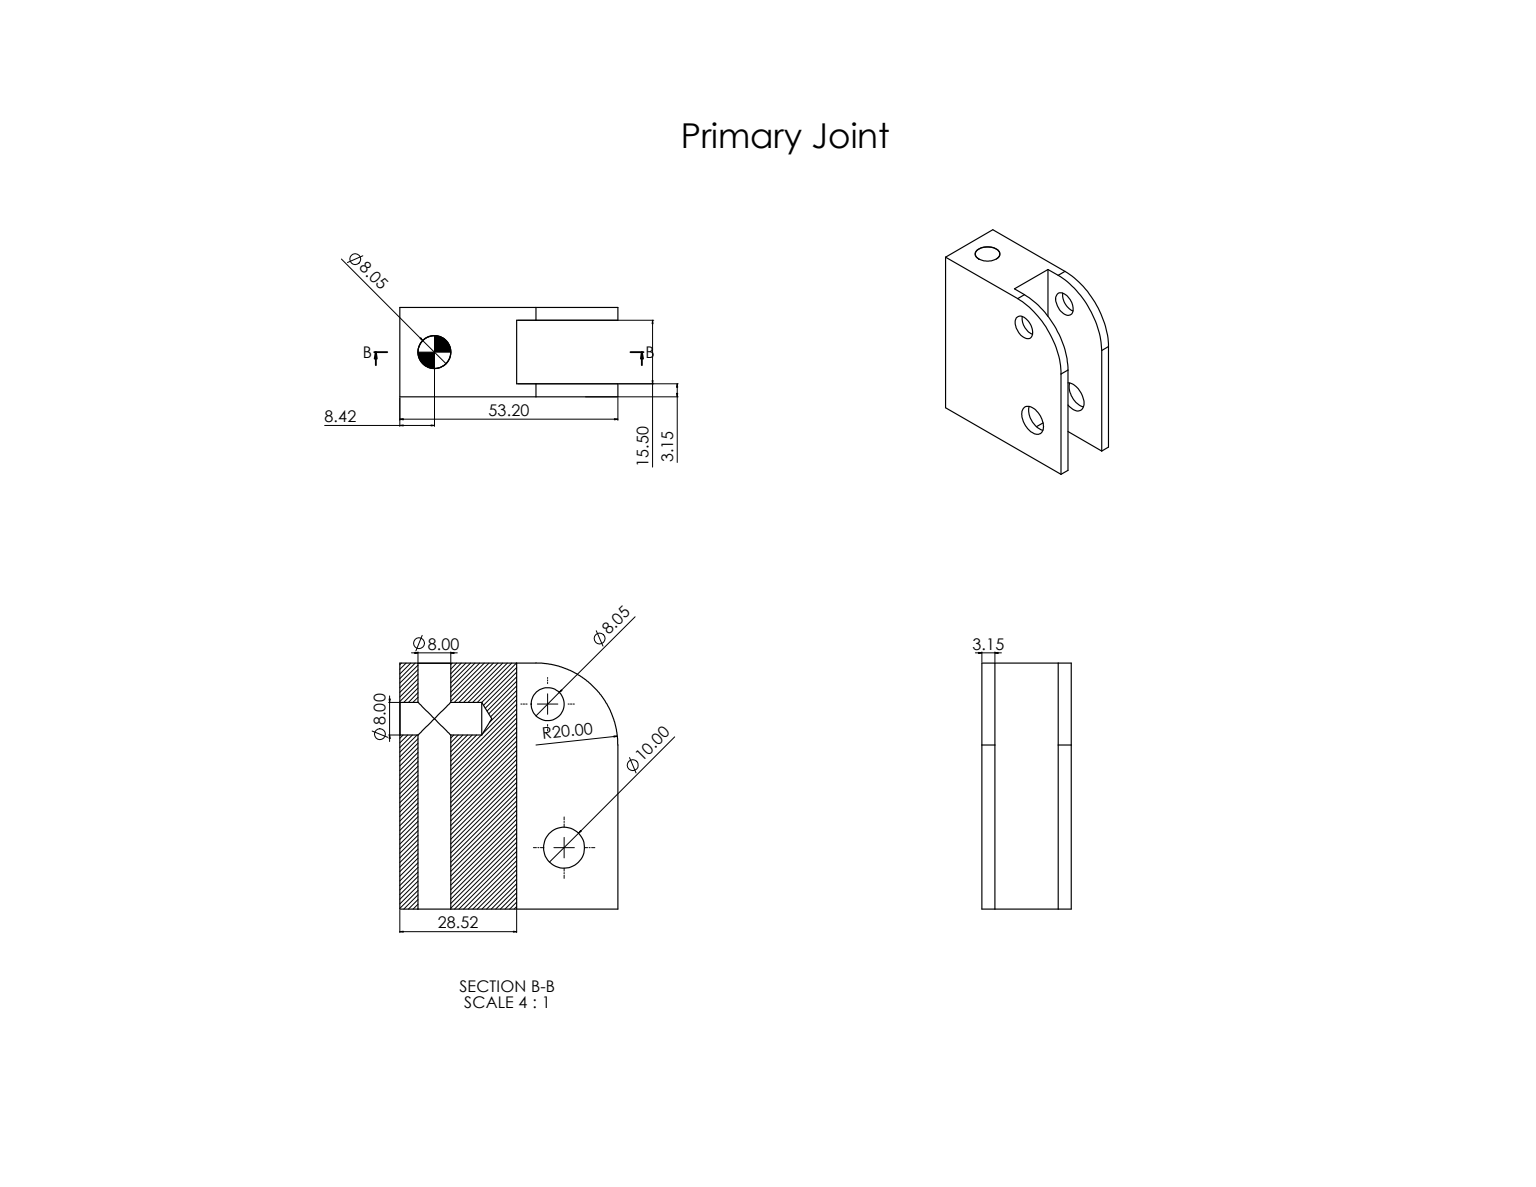
ISO-10303-21;
HEADER;
FILE_DESCRIPTION (('STEP AP214'),
    '1' );
FILE_NAME ('Primary Joint.step',
    '2026-10-20T14:49:59',
    ( '' ),
    ( '' ),
    'SwSTEP 2.0',
    'SolidWorks 2025',
    '' );
FILE_SCHEMA (( 'AUTOMOTIVE_DESIGN' ));
ENDSEC;

DATA;
#6=ORIENTED_EDGE ( 'NONE', *, *, #7618, .F. ) ;
#9=ORIENTED_EDGE ( 'NONE', *, *, #9037, .T. ) ;
#11=CARTESIAN_POINT ( 'NONE',  ( -47.94539818030330025, 137.0132282531173473, 3.999999999999991562 ) ) ;
#12=DIRECTION ( 'NONE',  ( 0.000000000000000000, 0.000000000000000000, 1.000000000000000000 ) ) ;
#20=ORIENTED_EDGE ( 'NONE', *, *, #4444, .T. ) ;
#26=AXIS2_PLACEMENT_3D ( 'NONE', #141, #5845, #6542 ) ;
#28=VECTOR ( 'NONE', #9785, 1000.000000000000000 ) ;
#38=AXIS2_PLACEMENT_3D ( 'NONE', #7742, #2701, #6091 ) ;
#50=DIRECTION ( 'NONE',  ( 1.000000000000000000, 0.000000000000000000, -1.734723475976805615E-16 ) ) ;
#62=ORIENTED_EDGE ( 'NONE', *, *, #3204, .F. ) ;
#63=CARTESIAN_POINT ( 'NONE',  ( -47.94539818030330025, 150.5696653505793563, 3.999999999999993339 ) ) ;
#68=CIRCLE ( 'NONE', #1421, 4.025000000000000355 ) ;
#84=VERTEX_POINT ( 'NONE', #3844 ) ;
#85=DIRECTION ( 'NONE',  ( 0.000000000000000000, 0.000000000000000000, -1.000000000000000000 ) ) ;
#96=DIRECTION ( 'NONE',  ( 0.000000000000000000, 0.000000000000000000, 1.000000000000000000 ) ) ;
#122=ORIENTED_EDGE ( 'NONE', *, *, #3348, .T. ) ;
#134=CIRCLE ( 'NONE', #4024, 3.999999999999993339 ) ;
#140=ORIENTED_EDGE ( 'NONE', *, *, #5070, .F. ) ;
#141=CARTESIAN_POINT ( 'NONE',  ( -23.17384457509314899, 130.5696653505793847, 10.90000000000000036 ) ) ;
#148=FACE_OUTER_BOUND ( 'NONE', #7245, .T. ) ;
#154=AXIS2_PLACEMENT_3D ( 'NONE', #9604, #3022, #736 ) ;
#166=CONICAL_SURFACE ( 'NONE', #1514, 4.025000000000000355, 0.7853981633977258348 ) ;
#168=ADVANCED_FACE ( 'NONE', ( #10363, #4632, #9677 ), #1511, .F. ) ;
#217=ORIENTED_EDGE ( 'NONE', *, *, #8260, .F. ) ;
#231=ORIENTED_EDGE ( 'NONE', *, *, #934, .T. ) ;
#236=DIRECTION ( 'NONE',  ( -1.000000000000000000, 0.000000000000000000, 9.101836848464096770E-17 ) ) ;
#240=EDGE_CURVE ( 'NONE', #10167, #8252, #4254, .T. ) ;
#245=CIRCLE ( 'NONE', #4296, 4.024999999999997691 ) ;
#250=AXIS2_PLACEMENT_3D ( 'NONE', #3199, #920, #4939 ) ;
#254=CARTESIAN_POINT ( 'NONE',  ( -56.36957570605427748, 150.5696653505793563, 10.90000000000000036 ) ) ;
#276=CARTESIAN_POINT ( 'NONE',  ( -21.29350689640810046, 105.5289575273812233, -25.04213562373096380 ) ) ;
#277=AXIS2_PLACEMENT_3D ( 'NONE', #10005, #5118, #7559 ) ;
#281=CARTESIAN_POINT ( 'NONE',  ( -27.85255513972543895, 150.5696653505793563, -7.749999999999996447 ) ) ;
#286=SHAPE_REPRESENTATION ( 'Primary Joint', ( #4601 ), #409 ) ;
#325=AXIS2_PLACEMENT_3D ( 'NONE', #7109, #9549, #7950 ) ;
#331=LINE ( 'NONE', #7790, #7501 ) ;
#343=DIRECTION ( 'NONE',  ( 1.000000000000000000, 0.000000000000000000, -9.101836848464095537E-17 ) ) ;
#350=CARTESIAN_POINT ( 'NONE',  ( -3.173844575093148990, 90.52895752738122326, -7.750000000000000000 ) ) ;
#360=DIRECTION ( 'NONE',  ( -0.000000000000000000, 1.000000000000000000, -0.000000000000000000 ) ) ;
#361=EDGE_LOOP ( 'NONE', ( #8543, #5301 ) ) ;
#374=VECTOR ( 'NONE', #4417, 1000.000000000000000 ) ;
#380=DIRECTION ( 'NONE',  ( -9.101836848464095537E-17, -0.000000000000000000, -1.000000000000000000 ) ) ;
#382=VERTEX_POINT ( 'NONE', #6794 ) ;
#386=AXIS2_PLACEMENT_3D ( 'NONE', #4274, #4902, #96 ) ;
#397=ORIENTED_EDGE ( 'NONE', *, *, #981, .F. ) ;
#404=LINE ( 'NONE', #3533, #7016 ) ;
#407=ORIENTED_EDGE ( 'NONE', *, *, #2639, .F. ) ;
#409=( GEOMETRIC_REPRESENTATION_CONTEXT ( 3 ) GLOBAL_UNCERTAINTY_ASSIGNED_CONTEXT ( ( #7381 ) ) GLOBAL_UNIT_ASSIGNED_CONTEXT ( ( #5955, #7452, #1930 ) ) REPRESENTATION_CONTEXT ( 'NONE', 'WORKASPACE' ) );
#435=CARTESIAN_POINT ( 'NONE',  ( -20.29350689640809691, 140.5696653505793563, -7.749999999999996447 ) ) ;
#445=FACE_OUTER_BOUND ( 'NONE', #4657, .T. ) ;
#459=VECTOR ( 'NONE', #2787, 1000.000000000000000 ) ;
#474=FACE_OUTER_BOUND ( 'NONE', #5248, .T. ) ;
#502=AXIS2_PLACEMENT_3D ( 'NONE', #2591, #6613, #4182 ) ;
#518=DIRECTION ( 'NONE',  ( -0.000000000000000000, 0.000000000000000000, -1.000000000000000000 ) ) ;
#526=PLANE ( 'NONE',  #8406 ) ;
#537=ORIENTED_EDGE ( 'NONE', *, *, #5206, .F. ) ;
#571=ORIENTED_EDGE ( 'NONE', *, *, #1163, .T. ) ;
#593=ORIENTED_EDGE ( 'NONE', *, *, #10466, .T. ) ;
#605=ADVANCED_FACE ( 'NONE', ( #5619 ), #1444, .F. ) ;
#610=DIRECTION ( 'NONE',  ( 0.000000000000000000, 1.000000000000000000, 0.000000000000000000 ) ) ;
#613=ORIENTED_EDGE ( 'NONE', *, *, #690, .T. ) ;
#614=CARTESIAN_POINT ( 'NONE',  ( -47.94539818030330025, 150.5696653505793563, 4.025000000000000355 ) ) ;
#615=EDGE_CURVE ( 'NONE', #2082, #4136, #3892, .T. ) ;
#623=VERTEX_POINT ( 'NONE', #3349 ) ;
#646=APPLICATION_CONTEXT ( 'automotive_design' ) ;
#661=ORIENTED_EDGE ( 'NONE', *, *, #1974, .F. ) ;
#665=LINE ( 'NONE', #3847, #1646 ) ;
#677=EDGE_CURVE ( 'NONE', #4096, #6235, #1697, .T. ) ;
#684=EDGE_LOOP ( 'NONE', ( #10046, #2690, #7813, #7655 ) ) ;
#690=EDGE_CURVE ( 'NONE', #1644, #4219, #1648, .T. ) ;
#691=EDGE_CURVE ( 'NONE', #1746, #382, #7319, .T. ) ;
#692=FACE_OUTER_BOUND ( 'NONE', #7714, .T. ) ;
#697=EDGE_LOOP ( 'NONE', ( #5887, #6931, #9069, #397 ) ) ;
#699=CARTESIAN_POINT ( 'NONE',  ( -36.36957570605426326, 137.0132282531173473, 4.000000000000003553 ) ) ;
#703=DIRECTION ( 'NONE',  ( 1.000000000000000000, 0.000000000000000000, 0.000000000000000000 ) ) ;
#725=LINE ( 'NONE', #4650, #5911 ) ;
#729=CARTESIAN_POINT ( 'NONE',  ( -20.29350689640809691, 140.5696653505793563, 10.90000000000000036 ) ) ;
#736=DIRECTION ( 'NONE',  ( 1.000000000000000000, 0.000000000000000000, 0.000000000000000000 ) ) ;
#744=EDGE_CURVE ( 'NONE', #623, #6132, #1660, .T. ) ;
#769=AXIS2_PLACEMENT_3D ( 'NONE', #8126, #4104, #6540 ) ;
#785=CARTESIAN_POINT ( 'NONE',  ( -3.173844575093148990, 90.52895752738122326, -10.90000000000000036 ) ) ;
#805=EDGE_CURVE ( 'NONE', #4824, #2551, #1327, .T. ) ;
#807=ORIENTED_EDGE ( 'NONE', *, *, #5966, .T. ) ;
#808=DIRECTION ( 'NONE',  ( -1.000000000000000000, 0.000000000000000000, 8.673617379884035472E-17 ) ) ;
#821=LINE ( 'NONE', #4057, #7300 ) ;
#840=CARTESIAN_POINT ( 'NONE',  ( -56.36957570605426326, 90.52895752738122326, -10.90000000000000036 ) ) ;
#841=DIRECTION ( 'NONE',  ( -9.101836848464095537E-17, -0.000000000000000000, -1.000000000000000000 ) ) ;
#854=EDGE_LOOP ( 'NONE', ( #9526, #8200, #20, #9001 ) ) ;
#866=STYLED_ITEM('',(#10532),#9943);
#868=EDGE_CURVE ( 'NONE', #10419, #3877, #1219, .T. ) ;
#877=CARTESIAN_POINT ( 'NONE',  ( -20.29350689640809691, 140.5696653505793563, 10.90000000000000036 ) ) ;
#879=CARTESIAN_POINT ( 'NONE',  ( -11.29350689640809158, 105.5289575273812233, -10.90000000000000036 ) ) ;
#887=LINE ( 'NONE', #2642, #9640 ) ;
#894=EDGE_CURVE ( 'NONE', #8252, #3355, #2912, .T. ) ;
#897=ORIENTED_EDGE ( 'NONE', *, *, #8642, .F. ) ;
#907=VECTOR ( 'NONE', #3811, 1000.000000000000000 ) ;
#920=DIRECTION ( 'NONE',  ( 1.137729606058012035E-16, 0.000000000000000000, 1.000000000000000000 ) ) ;
#923=ORIENTED_EDGE ( 'NONE', *, *, #5411, .F. ) ;
#934=EDGE_CURVE ( 'NONE', #8880, #7785, #4717, .T. ) ;
#950=CARTESIAN_POINT ( 'NONE',  ( -56.36957570605427748, 150.5696653505793563, -10.90000000000000036 ) ) ;
#960=CARTESIAN_POINT ( 'NONE',  ( -47.94539818030330025, 150.5446653505793790, -3.999999999999989786 ) ) ;
#981=EDGE_CURVE ( 'NONE', #2288, #3945, #9975, .T. ) ;
#1000=DIRECTION ( 'NONE',  ( -0.000000000000000000, -0.000000000000000000, -1.000000000000000000 ) ) ;
#1004=ORIENTED_EDGE ( 'NONE', *, *, #6311, .T. ) ;
#1053=EDGE_CURVE ( 'NONE', #8741, #6235, #5555, .T. ) ;
#1112=CARTESIAN_POINT ( 'NONE',  ( -36.36957570605426326, 137.0132282531173473, 0.000000000000000000 ) ) ;
#1126=DIRECTION ( 'NONE',  ( -1.000000000000000000, -0.000000000000000000, -0.000000000000000000 ) ) ;
#1129=LINE ( 'NONE', #1765, #4999 ) ;
#1163=EDGE_CURVE ( 'NONE', #6235, #6817, #1738, .T. ) ;
#1166=VERTEX_POINT ( 'NONE', #785 ) ;
#1192=CYLINDRICAL_SURFACE ( 'NONE', #6034, 20.00000000000000000 ) ;
#1195=DIRECTION ( 'NONE',  ( 0.000000000000000000, -1.000000000000000000, 0.000000000000000000 ) ) ;
#1200=EDGE_CURVE ( 'NONE', #7910, #7087, #887, .T. ) ;
#1201=ORIENTED_EDGE ( 'NONE', *, *, #1675, .T. ) ;
#1210=CARTESIAN_POINT ( 'NONE',  ( -27.85255513972543895, 150.5696653505793563, 7.750000000000002665 ) ) ;
#1219=LINE ( 'NONE', #276, #5717 ) ;
#1230=EDGE_LOOP ( 'NONE', ( #6888, #8370, #3768, #8353 ) ) ;
#1243=EDGE_CURVE ( 'NONE', #1644, #2082, #5896, .T. ) ;
#1289=LINE ( 'NONE', #10253, #8564 ) ;
#1319=DIRECTION ( 'NONE',  ( 1.000000000000000000, 0.000000000000000000, -0.000000000000000000 ) ) ;
#1324=EDGE_CURVE ( 'NONE', #2102, #8741, #3648, .T. ) ;
#1327=LINE ( 'NONE', #9223, #1666 ) ;
#1336=EDGE_CURVE ( 'NONE', #8252, #7910, #7889, .T. ) ;
#1347=ORIENTED_EDGE ( 'NONE', *, *, #1675, .F. ) ;
#1357=ORIENTED_EDGE ( 'NONE', *, *, #2172, .F. ) ;
#1369=DIRECTION ( 'NONE',  ( 1.000000000000000000, 0.000000000000000000, 0.000000000000000000 ) ) ;
#1372=CARTESIAN_POINT ( 'NONE',  ( -33.96613322994402751, 137.0132282531173473, 0.000000000000000000 ) ) ;
#1391=CARTESIAN_POINT ( 'NONE',  ( -56.36957570605427037, 137.0132282531173473, 0.000000000000000000 ) ) ;
#1393=LINE ( 'NONE', #3729, #6363 ) ;
#1421=AXIS2_PLACEMENT_3D ( 'NONE', #9108, #7361, #5075 ) ;
#1427=EDGE_CURVE ( 'NONE', #5184, #10246, #5343, .T. ) ;
#1428=ORIENTED_EDGE ( 'NONE', *, *, #6311, .F. ) ;
#1435=DIRECTION ( 'NONE',  ( -3.081165567444019513E-16, 1.000000000000000000, 0.000000000000000000 ) ) ;
#1436=DIRECTION ( 'NONE',  ( -0.000000000000000000, -0.000000000000000000, 1.000000000000000000 ) ) ;
#1444=CYLINDRICAL_SURFACE ( 'NONE', #9626, 3.999999999999989786 ) ;
#1445=DIRECTION ( 'NONE',  ( -0.000000000000000000, 1.000000000000000000, -0.000000000000000000 ) ) ;
#1453=EDGE_CURVE ( 'NONE', #10419, #9834, #8224, .T. ) ;
#1457=DIRECTION ( 'NONE',  ( 1.137729606058012035E-16, 0.000000000000000000, 1.000000000000000000 ) ) ;
#1458=AXIS2_PLACEMENT_3D ( 'NONE', #9422, #3108, #10330 ) ;
#1464=ORIENTED_EDGE ( 'NONE', *, *, #8642, .T. ) ;
#1466=VECTOR ( 'NONE', #6032, 1000.000000000000000 ) ;
#1467=EDGE_LOOP ( 'NONE', ( #2773, #217, #5935, #2397 ) ) ;
#1477=DIRECTION ( 'NONE',  ( -0.000000000000000000, -0.000000000000000000, 1.000000000000000000 ) ) ;
#1508=CARTESIAN_POINT ( 'NONE',  ( -16.29350689640809691, 105.5289575273812233, -25.04213562373096380 ) ) ;
#1510=ORIENTED_EDGE ( 'NONE', *, *, #3911, .F. ) ;
#1511=PLANE ( 'NONE',  #6559 ) ;
#1514=AXIS2_PLACEMENT_3D ( 'NONE', #2760, #5991, #9233 ) ;
#1519=CARTESIAN_POINT ( 'NONE',  ( -16.26850689640809833, 140.5696653505793563, -7.749999999999996447 ) ) ;
#1522=CARTESIAN_POINT ( 'NONE',  ( -47.94539818030330025, 150.5696653505793563, 0.000000000000000000 ) ) ;
#1535=VERTEX_POINT ( 'NONE', #7884 ) ;
#1536=DIRECTION ( 'NONE',  ( -1.000000000000000000, -0.000000000000000000, -0.000000000000000000 ) ) ;
#1554=EDGE_CURVE ( 'NONE', #10167, #5689, #1129, .T. ) ;
#1558=SHAPE_REPRESENTATION_RELATIONSHIP ( 'NONE' , 'NONE' ,  #286, #5432 ) ;
#1560=AXIS2_PLACEMENT_3D ( 'NONE', #7664, #360, #6926 ) ;
#1564=DIRECTION ( 'NONE',  ( -0.000000000000000000, 1.000000000000000000, -0.000000000000000000 ) ) ;
#1566=EDGE_LOOP ( 'NONE', ( #5795, #7193, #8868, #923 ) ) ;
#1568=DIRECTION ( 'NONE',  ( 0.000000000000000000, 0.000000000000000000, 1.000000000000000000 ) ) ;
#1570=EDGE_LOOP ( 'NONE', ( #231, #4645 ) ) ;
#1588=CARTESIAN_POINT ( 'NONE',  ( -16.29350689640809691, 105.5289575273812233, -25.04213562373096380 ) ) ;
#1610=LINE ( 'NONE', #9729, #10068 ) ;
#1621=DIRECTION ( 'NONE',  ( -0.000000000000000000, -0.000000000000000000, -1.000000000000000000 ) ) ;
#1630=CARTESIAN_POINT ( 'NONE',  ( -27.85255513972543895, 150.5696653505793563, 7.750000000000002665 ) ) ;
#1644=VERTEX_POINT ( 'NONE', #9993 ) ;
#1645=ORIENTED_EDGE ( 'NONE', *, *, #8978, .F. ) ;
#1646=VECTOR ( 'NONE', #7816, 1000.000000000000000 ) ;
#1648=LINE ( 'NONE', #3394, #2167 ) ;
#1660=CIRCLE ( 'NONE', #7585, 4.025000000000000355 ) ;
#1666=VECTOR ( 'NONE', #2803, 1000.000000000000000 ) ;
#1671=DIRECTION ( 'NONE',  ( 0.000000000000000000, 1.000000000000000000, 0.000000000000000000 ) ) ;
#1675=EDGE_CURVE ( 'NONE', #10069, #2784, #1393, .T. ) ;
#1678=DIRECTION ( 'NONE',  ( -0.5150380749100536004, 1.049727191138618942E-16, -0.8571673007021125557 ) ) ;
#1684=EDGE_LOOP ( 'NONE', ( #3521, #4698 ) ) ;
#1685=CARTESIAN_POINT ( 'NONE',  ( -16.29350689640809691, 105.5289575273812233, 7.750000000000000000 ) ) ;
#1689=DIRECTION ( 'NONE',  ( -0.000000000000000000, -0.000000000000000000, 1.000000000000000000 ) ) ;
#1697=LINE ( 'NONE', #8319, #3178 ) ;
#1717=VECTOR ( 'NONE', #85, 1000.000000000000000 ) ;
#1738=LINE ( 'NONE', #4127, #5048 ) ;
#1746=VERTEX_POINT ( 'NONE', #10143 ) ;
#1755=ORIENTED_EDGE ( 'NONE', *, *, #8260, .T. ) ;
#1764=( LENGTH_UNIT ( ) NAMED_UNIT ( * ) SI_UNIT ( .MILLI., .METRE. ) );
#1765=CARTESIAN_POINT ( 'NONE',  ( 10.26554134690924691, 150.5696653505793563, -7.750000000000000000 ) ) ;
#1771=CARTESIAN_POINT ( 'NONE',  ( -24.31850689640809549, 140.5696653505793563, -7.749999999999996447 ) ) ;
#1836=LINE ( 'NONE', #6554, #3429 ) ;
#1842=DIRECTION ( 'NONE',  ( 1.000000000000000000, -0.000000000000000000, -1.137729606058012035E-16 ) ) ;
#1852=EDGE_LOOP ( 'NONE', ( #897, #1347, #7000, #8533, #3240, #6980, #4738, #1854 ) ) ;
#1854=ORIENTED_EDGE ( 'NONE', *, *, #8258, .T. ) ;
#1890=DIRECTION ( 'NONE',  ( 0.000000000000000000, 0.000000000000000000, 1.000000000000000000 ) ) ;
#1902=EDGE_CURVE ( 'NONE', #2551, #1535, #6369, .T. ) ;
#1906=VECTOR ( 'NONE', #5257, 1000.000000000000000 ) ;
#1930=( NAMED_UNIT ( * ) SI_UNIT ( $, .STERADIAN. ) SOLID_ANGLE_UNIT ( ) );
#1974=EDGE_CURVE ( 'NONE', #6132, #623, #3668, .T. ) ;
#1976=EDGE_CURVE ( 'NONE', #6245, #7785, #10233, .T. ) ;
#1977=VECTOR ( 'NONE', #4423, 1000.000000000000000 ) ;
#1989=CARTESIAN_POINT ( 'NONE',  ( -23.17384457509314544, 150.5696653505793563, 7.750000000000001776 ) ) ;
#2008=ADVANCED_FACE ( 'NONE', ( #4603, #8474 ), #526, .F. ) ;
#2052=FACE_OUTER_BOUND ( 'NONE', #3019, .T. ) ;
#2060=ORIENTED_EDGE ( 'NONE', *, *, #9362, .T. ) ;
#2072=ORIENTED_EDGE ( 'NONE', *, *, #6556, .F. ) ;
#2082=VERTEX_POINT ( 'NONE', #7302 ) ;
#2083=CARTESIAN_POINT ( 'NONE',  ( -47.94539818030330025, 150.5696653505793563, -4.025000000000000355 ) ) ;
#2086=CARTESIAN_POINT ( 'NONE',  ( -23.17384457509314899, 130.5696653505793847, 10.90000000000000036 ) ) ;
#2102=VERTEX_POINT ( 'NONE', #1630 ) ;
#2112=FACE_BOUND ( 'NONE', #4060, .T. ) ;
#2126=VECTOR ( 'NONE', #3478, 1000.000000000000000 ) ;
#2143=CARTESIAN_POINT ( 'NONE',  ( -56.34457570605425758, 137.0132282531173473, 3.999999999999976019 ) ) ;
#2151=ORIENTED_EDGE ( 'NONE', *, *, #4357, .T. ) ;
#2167=VECTOR ( 'NONE', #9926, 1000.000000000000000 ) ;
#2172=EDGE_CURVE ( 'NONE', #10246, #382, #5558, .T. ) ;
#2183=ORIENTED_EDGE ( 'NONE', *, *, #744, .F. ) ;
#2198=CARTESIAN_POINT ( 'NONE',  ( -47.94539818030330025, 137.0132282531173473, -3.999999999999991562 ) ) ;
#2202=EDGE_LOOP ( 'NONE', ( #7733, #10267, #3875, #7881, #9652 ) ) ;
#2220=ORIENTED_EDGE ( 'NONE', *, *, #1243, .T. ) ;
#2231=VECTOR ( 'NONE', #1195, 1000.000000000000000 ) ;
#2234=ADVANCED_FACE ( 'NONE', ( #10010 ), #3329, .F. ) ;
#2258=CARTESIAN_POINT ( 'NONE',  ( -3.173844575093148990, 130.5696653505793847, 7.750000000000000000 ) ) ;
#2263=ORIENTED_EDGE ( 'NONE', *, *, #4916, .T. ) ;
#2269=AXIS2_PLACEMENT_3D ( 'NONE', #6346, #1477, #1369 ) ;
#2279=ORIENTED_EDGE ( 'NONE', *, *, #1200, .F. ) ;
#2283=CARTESIAN_POINT ( 'NONE',  ( -20.29350689640809691, 140.5696653505793563, 10.90000000000000036 ) ) ;
#2288=VERTEX_POINT ( 'NONE', #5015 ) ;
#2289=AXIS2_PLACEMENT_3D ( 'NONE', #4666, #5460, #10393 ) ;
#2307=PRODUCT ( 'Primary Joint', 'Primary Joint', '', ( #2315 ) ) ;
#2315=PRODUCT_CONTEXT ( 'NONE', #646, 'mechanical' ) ;
#2331=AXIS2_PLACEMENT_3D ( 'NONE', #7792, #7588, #7005 ) ;
#2338=DIRECTION ( 'NONE',  ( -1.000000000000000000, -0.000000000000000000, -0.000000000000000000 ) ) ;
#2345=VECTOR ( 'NONE', #5435, 1000.000000000000000 ) ;
#2374=ORIENTED_EDGE ( 'NONE', *, *, #981, .T. ) ;
#2375=DIRECTION ( 'NONE',  ( -1.137729606058012035E-16, -0.000000000000000000, -1.000000000000000000 ) ) ;
#2380=EDGE_LOOP ( 'NONE', ( #8279, #9, #5242, #2072 ) ) ;
#2383=ORIENTED_EDGE ( 'NONE', *, *, #1163, .F. ) ;
#2388=( GEOMETRIC_REPRESENTATION_CONTEXT ( 3 ) GLOBAL_UNCERTAINTY_ASSIGNED_CONTEXT ( ( #9833 ) ) GLOBAL_UNIT_ASSIGNED_CONTEXT ( ( #1764, #4099, #4255 ) ) REPRESENTATION_CONTEXT ( 'NONE', 'WORKASPACE' ) );
#2397=ORIENTED_EDGE ( 'NONE', *, *, #7618, .T. ) ;
#2407=EDGE_LOOP ( 'NONE', ( #8584, #3415 ) ) ;
#2442=AXIS2_PLACEMENT_3D ( 'NONE', #7793, #6693, #2618 ) ;
#2458=FACE_OUTER_BOUND ( 'NONE', #3220, .T. ) ;
#2467=DIRECTION ( 'NONE',  ( 0.000000000000000000, 0.000000000000000000, -1.000000000000000000 ) ) ;
#2468=LINE ( 'NONE', #5695, #4671 ) ;
#2473=EDGE_CURVE ( 'NONE', #1535, #5197, #7669, .T. ) ;
#2480=FACE_OUTER_BOUND ( 'NONE', #8443, .T. ) ;
#2494=CLOSED_SHELL ( 'NONE', ( #6615, #4121, #6110, #6557, #8776, #2563, #2234, #10016, #9921, #9641, #605, #7555, #2809, #8581, #9569, #6898, #4061, #9141, #8020, #2008, #8104, #10074, #168, #6055, #3671, #6423, #3511, #3092, #5918, #10464, #9230, #5878, #8436, #8217 ) ) ;
#2532=FACE_BOUND ( 'NONE', #361, .T. ) ;
#2533=CARTESIAN_POINT ( 'NONE',  ( -47.94539818030330025, 150.5446653505793790, 0.000000000000000000 ) ) ;
#2534=DIRECTION ( 'NONE',  ( 1.000000000000000000, 0.000000000000000000, 0.000000000000000000 ) ) ;
#2536=DIRECTION ( 'NONE',  ( 0.000000000000000000, 0.000000000000000000, 1.000000000000000000 ) ) ;
#2551=VERTEX_POINT ( 'NONE', #10325 ) ;
#2557=ORIENTED_EDGE ( 'NONE', *, *, #6529, .T. ) ;
#2563=ADVANCED_FACE ( 'NONE', ( #4644 ), #3208, .F. ) ;
#2591=CARTESIAN_POINT ( 'NONE',  ( -16.29350689640809691, 105.5289575273812233, -7.749999999999996447 ) ) ;
#2592=CARTESIAN_POINT ( 'NONE',  ( -16.29350689640809691, 105.5289575273812233, -25.04213562373096380 ) ) ;
#2612=PRODUCT_DEFINITION_CONTEXT ( 'detailed design', #9516, 'design' ) ;
#2618=DIRECTION ( 'NONE',  ( 0.000000000000000000, -0.000000000000000000, -1.000000000000000000 ) ) ;
#2624=AXIS2_PLACEMENT_3D ( 'NONE', #2645, #4074, #5076 ) ;
#2639=EDGE_CURVE ( 'NONE', #3419, #623, #7291, .T. ) ;
#2642=CARTESIAN_POINT ( 'NONE',  ( -3.173844575093148990, 130.5696653505793847, 10.90000000000000036 ) ) ;
#2645=CARTESIAN_POINT ( 'NONE',  ( -56.34457570605425758, 137.0132282531173473, 0.000000000000000000 ) ) ;
#2655=CARTESIAN_POINT ( 'NONE',  ( -24.31850689640809549, 140.5696653505793563, 7.750000000000002665 ) ) ;
#2663=VERTEX_POINT ( 'NONE', #5690 ) ;
#2683=CARTESIAN_POINT ( 'NONE',  ( -23.17384457509314899, 150.5696653505793563, 10.90000000000000036 ) ) ;
#2685=DIRECTION ( 'NONE',  ( -1.000000000000000000, 0.000000000000000000, 0.000000000000000000 ) ) ;
#2686=DIRECTION ( 'NONE',  ( -0.7071067811863512853, 0.000000000000000000, 0.7071067811867437491 ) ) ;
#2690=ORIENTED_EDGE ( 'NONE', *, *, #9935, .T. ) ;
#2695=CARTESIAN_POINT ( 'NONE',  ( -11.29350689640809158, 105.5289575273812233, -7.749999999999997335 ) ) ;
#2701=DIRECTION ( 'NONE',  ( -0.000000000000000000, -1.000000000000000000, -0.000000000000000000 ) ) ;
#2747=AXIS2_PLACEMENT_3D ( 'NONE', #4484, #6070, #10007 ) ;
#2760=CARTESIAN_POINT ( 'NONE',  ( -47.94539818030330025, 150.5696653505793563, 0.000000000000000000 ) ) ;
#2773=ORIENTED_EDGE ( 'NONE', *, *, #9575, .F. ) ;
#2775=DIRECTION ( 'NONE',  ( -1.000000000000000000, 0.000000000000000000, 0.000000000000000000 ) ) ;
#2784=VERTEX_POINT ( 'NONE', #350 ) ;
#2787=DIRECTION ( 'NONE',  ( 1.000000000000000000, 0.000000000000000000, -0.000000000000000000 ) ) ;
#2794=DIRECTION ( 'NONE',  ( -0.000000000000000000, 1.000000000000000000, -0.000000000000000000 ) ) ;
#2798=EDGE_LOOP ( 'NONE', ( #10043, #9182, #5890, #1464 ) ) ;
#2803=DIRECTION ( 'NONE',  ( -1.000000000000000000, 0.000000000000000000, 0.000000000000000000 ) ) ;
#2809=ADVANCED_FACE ( 'NONE', ( #4376 ), #5951, .F. ) ;
#2822=CIRCLE ( 'NONE', #9606, 20.00000000000000000 ) ;
#2827=DIRECTION ( 'NONE',  ( -0.000000000000000000, 0.000000000000000000, -1.000000000000000000 ) ) ;
#2838=PLANE ( 'NONE',  #2747 ) ;
#2856=ORIENTED_EDGE ( 'NONE', *, *, #8978, .T. ) ;
#2861=CIRCLE ( 'NONE', #10326, 3.999999999999989786 ) ;
#2864=ORIENTED_EDGE ( 'NONE', *, *, #3131, .T. ) ;
#2903=DIRECTION ( 'NONE',  ( 0.000000000000000000, 0.000000000000000000, 1.000000000000000000 ) ) ;
#2904=DIRECTION ( 'NONE',  ( -0.5150380749100536004, 0.000000000000000000, 0.8571673007021125557 ) ) ;
#2912=LINE ( 'NONE', #10024, #9458 ) ;
#2918=FACE_OUTER_BOUND ( 'NONE', #2931, .T. ) ;
#2920=ORIENTED_EDGE ( 'NONE', *, *, #8790, .F. ) ;
#2922=AXIS2_PLACEMENT_3D ( 'NONE', #6002, #9300, #3572 ) ;
#2924=ORIENTED_EDGE ( 'NONE', *, *, #9575, .T. ) ;
#2930=DIRECTION ( 'NONE',  ( 0.000000000000000000, 0.000000000000000000, 1.000000000000000000 ) ) ;
#2931=EDGE_LOOP ( 'NONE', ( #6718, #3471, #9051, #5950, #3891, #8620, #7163, #8412 ) ) ;
#2950=ORIENTED_EDGE ( 'NONE', *, *, #744, .T. ) ;
#2994=CARTESIAN_POINT ( 'NONE',  ( -3.173844575093148990, 105.5289575273812233, -10.90000000000000036 ) ) ;
#3008=EDGE_CURVE ( 'NONE', #10256, #7686, #3192, .T. ) ;
#3019=EDGE_LOOP ( 'NONE', ( #7704, #6448, #613, #6936 ) ) ;
#3022=DIRECTION ( 'NONE',  ( 0.000000000000000000, 0.000000000000000000, 1.000000000000000000 ) ) ;
#3041=DIRECTION ( 'NONE',  ( 0.000000000000000000, 0.000000000000000000, 1.000000000000000000 ) ) ;
#3045=DIRECTION ( 'NONE',  ( 0.000000000000000000, 0.000000000000000000, -1.000000000000000000 ) ) ;
#3071=CYLINDRICAL_SURFACE ( 'NONE', #4289, 4.024999999999997691 ) ;
#3084=ORIENTED_EDGE ( 'NONE', *, *, #2639, .T. ) ;
#3092=ADVANCED_FACE ( 'NONE', ( #6788 ), #166, .F. ) ;
#3093=EDGE_LOOP ( 'NONE', ( #1645, #6402, #5095, #7331 ) ) ;
#3102=CIRCLE ( 'NONE', #10214, 4.024999999999997691 ) ;
#3108=DIRECTION ( 'NONE',  ( -1.000000000000000000, -0.000000000000000000, -0.000000000000000000 ) ) ;
#3129=ORIENTED_EDGE ( 'NONE', *, *, #3719, .F. ) ;
#3131=EDGE_CURVE ( 'NONE', #9513, #5509, #2861, .T. ) ;
#3178=VECTOR ( 'NONE', #9822, 1000.000000000000000 ) ;
#3192=LINE ( 'NONE', #9672, #7264 ) ;
#3196=EDGE_LOOP ( 'NONE', ( #9370, #5836, #6636, #8156, #7720 ) ) ;
#3199=CARTESIAN_POINT ( 'NONE',  ( -16.29350689640809691, 105.5289575273812233, 7.750000000000000000 ) ) ;
#3204=EDGE_CURVE ( 'NONE', #3877, #4343, #9651, .T. ) ;
#3208=CYLINDRICAL_SURFACE ( 'NONE', #9807, 3.999999999999993339 ) ;
#3215=FACE_OUTER_BOUND ( 'NONE', #9314, .T. ) ;
#3220=EDGE_LOOP ( 'NONE', ( #7142, #2279, #8423, #6831 ) ) ;
#3240=ORIENTED_EDGE ( 'NONE', *, *, #8119, .F. ) ;
#3243=CONICAL_SURFACE ( 'NONE', #6635, 4.000000000000003553, 1.029744258676655200 ) ;
#3258=DIRECTION ( 'NONE',  ( -0.000000000000000000, 1.000000000000000000, -0.000000000000000000 ) ) ;
#3271=FACE_OUTER_BOUND ( 'NONE', #4514, .T. ) ;
#3274=AXIS2_PLACEMENT_3D ( 'NONE', #10018, #5180, #7626 ) ;
#3280=DIRECTION ( 'NONE',  ( -1.000000000000000000, 0.000000000000000000, 1.734723475976805615E-16 ) ) ;
#3292=DIRECTION ( 'NONE',  ( -0.000000000000000000, -1.000000000000000000, -0.000000000000000000 ) ) ;
#3293=ORIENTED_EDGE ( 'NONE', *, *, #5347, .F. ) ;
#3323=CARTESIAN_POINT ( 'NONE',  ( -47.94539818030330025, 150.5696653505793563, 0.000000000000000000 ) ) ;
#3329=CONICAL_SURFACE ( 'NONE', #4520, 4.025000000000000355, 0.7853981633977258348 ) ;
#3336=DIRECTION ( 'NONE',  ( 0.000000000000000000, 0.000000000000000000, 1.000000000000000000 ) ) ;
#3338=DIRECTION ( 'NONE',  ( -1.000000000000000000, -0.000000000000000000, -0.000000000000000000 ) ) ;
#3348=EDGE_CURVE ( 'NONE', #6390, #8880, #725, .T. ) ;
#3349=CARTESIAN_POINT ( 'NONE',  ( -56.36957570605427037, 137.0132282531173473, -4.025000000000000355 ) ) ;
#3355=VERTEX_POINT ( 'NONE', #6289 ) ;
#3393=VERTEX_POINT ( 'NONE', #9481 ) ;
#3394=CARTESIAN_POINT ( 'NONE',  ( -11.29350689640809158, 105.5289575273812233, -25.04213562373096380 ) ) ;
#3412=CARTESIAN_POINT ( 'NONE',  ( -36.36957570605426326, 137.0132282531173473, -4.000000000000003553 ) ) ;
#3415=ORIENTED_EDGE ( 'NONE', *, *, #6587, .F. ) ;
#3419=VERTEX_POINT ( 'NONE', #5442 ) ;
#3429=VECTOR ( 'NONE', #2686, 1000.000000000000000 ) ;
#3431=DIRECTION ( 'NONE',  ( -0.000000000000000000, 1.000000000000000000, -0.000000000000000000 ) ) ;
#3437=DIRECTION ( 'NONE',  ( 0.000000000000000000, 0.000000000000000000, -1.000000000000000000 ) ) ;
#3470=CIRCLE ( 'NONE', #3818, 5.000000000000004441 ) ;
#3471=ORIENTED_EDGE ( 'NONE', *, *, #6433, .T. ) ;
#3478=DIRECTION ( 'NONE',  ( -0.000000000000000000, -0.000000000000000000, -1.000000000000000000 ) ) ;
#3482=ORIENTED_EDGE ( 'NONE', *, *, #2473, .T. ) ;
#3487=CARTESIAN_POINT ( 'NONE',  ( -3.173844575093148990, 130.5696653505793847, -7.750000000000000000 ) ) ;
#3490=CYLINDRICAL_SURFACE ( 'NONE', #3789, 5.000000000000004441 ) ;
#3492=AXIS2_PLACEMENT_3D ( 'NONE', #7019, #2930, #703 ) ;
#3511=ADVANCED_FACE ( 'NONE', ( #148 ), #8243, .F. ) ;
#3521=ORIENTED_EDGE ( 'NONE', *, *, #7956, .T. ) ;
#3522=LINE ( 'NONE', #2083, #374 ) ;
#3533=CARTESIAN_POINT ( 'NONE',  ( -27.85255513972543895, 64.37996872128307757, -7.749999999999996447 ) ) ;
#3535=DIRECTION ( 'NONE',  ( -0.000000000000000000, -0.000000000000000000, -1.000000000000000000 ) ) ;
#3555=EDGE_LOOP ( 'NONE', ( #4070, #8995, #4266 ) ) ;
#3572=DIRECTION ( 'NONE',  ( 0.000000000000000000, 0.000000000000000000, 1.000000000000000000 ) ) ;
#3591=( BOUNDED_CURVE ( )  B_SPLINE_CURVE ( 3, ( #10457, #6268, #7125, #7272 ),
 .UNSPECIFIED., .F., .T. ) 
 B_SPLINE_CURVE_WITH_KNOTS ( ( 4, 4 ),
 ( 1.570796326794896558, 4.712388980384689674 ),
 .UNSPECIFIED. ) 
 CURVE ( )  GEOMETRIC_REPRESENTATION_ITEM ( )  RATIONAL_B_SPLINE_CURVE ( ( 1.000000000000000000, 0.3333333333333333703, 0.3333333333333333703, 1.000000000000000000 ) ) 
 REPRESENTATION_ITEM ( '' )  );
#3597=EDGE_CURVE ( 'NONE', #382, #9513, #5853, .T. ) ;
#3621=CARTESIAN_POINT ( 'NONE',  ( 10.26554134690924691, 64.37996872128307757, -7.750000000000000000 ) ) ;
#3648=LINE ( 'NONE', #10118, #7053 ) ;
#3663=DIRECTION ( 'NONE',  ( -0.000000000000000000, -0.000000000000000000, 1.000000000000000000 ) ) ;
#3668=CIRCLE ( 'NONE', #7062, 4.025000000000000355 ) ;
#3671=ADVANCED_FACE ( 'NONE', ( #8453 ), #1192, .T. ) ;
#3683=CARTESIAN_POINT ( 'NONE',  ( -55.94539818030328604, 129.0132282531173757, 3.999999999999992895 ) ) ;
#3693=DIRECTION ( 'NONE',  ( -1.000000000000000000, -0.000000000000000000, -0.000000000000000000 ) ) ;
#3696=ORIENTED_EDGE ( 'NONE', *, *, #3008, .F. ) ;
#3698=ORIENTED_EDGE ( 'NONE', *, *, #1554, .T. ) ;
#3709=PLANE ( 'NONE',  #4079 ) ;
#3712=ORIENTED_EDGE ( 'NONE', *, *, #1976, .F. ) ;
#3716=CARTESIAN_POINT ( 'NONE',  ( -21.29350689640810046, 105.5289575273812233, -10.90000000000000036 ) ) ;
#3719=EDGE_CURVE ( 'NONE', #9834, #4343, #665, .T. ) ;
#3728=CARTESIAN_POINT ( 'NONE',  ( -56.36957570605427037, 137.0132282531173473, 0.000000000000000000 ) ) ;
#3729=CARTESIAN_POINT ( 'NONE',  ( 10.26554134690924691, 90.52895752738122326, -7.750000000000000000 ) ) ;
#3733=EDGE_CURVE ( 'NONE', #1166, #7910, #10259, .T. ) ;
#3748=AXIS2_PLACEMENT_3D ( 'NONE', #3621, #9344, #8386 ) ;
#3761=EDGE_CURVE ( 'NONE', #7686, #382, #6428, .T. ) ;
#3768=ORIENTED_EDGE ( 'NONE', *, *, #7706, .T. ) ;
#3772=ORIENTED_EDGE ( 'NONE', *, *, #8402, .F. ) ;
#3789=AXIS2_PLACEMENT_3D ( 'NONE', #2592, #1689, #2534 ) ;
#3811=DIRECTION ( 'NONE',  ( 0.000000000000000000, 0.7071067811863512853, 0.7071067811867437491 ) ) ;
#3818=AXIS2_PLACEMENT_3D ( 'NONE', #5760, #841, #3280 ) ;
#3835=FACE_OUTER_BOUND ( 'NONE', #1230, .T. ) ;
#3844=CARTESIAN_POINT ( 'NONE',  ( -24.31850689640809549, 140.5696653505793563, 10.90000000000000036 ) ) ;
#3847=CARTESIAN_POINT ( 'NONE',  ( -11.29350689640809158, 105.5289575273812233, -25.04213562373096380 ) ) ;
#3875=ORIENTED_EDGE ( 'NONE', *, *, #677, .F. ) ;
#3877=VERTEX_POINT ( 'NONE', #5931 ) ;
#3891=ORIENTED_EDGE ( 'NONE', *, *, #1554, .F. ) ;
#3892=LINE ( 'NONE', #8855, #7244 ) ;
#3899=CARTESIAN_POINT ( 'NONE',  ( -27.85255513972543895, 90.52895752738122326, 7.750000000000002665 ) ) ;
#3911=EDGE_CURVE ( 'NONE', #10256, #1746, #134, .T. ) ;
#3929=CARTESIAN_POINT ( 'NONE',  ( -56.36957570605427748, 150.5696653505793563, 10.90000000000000036 ) ) ;
#3932=AXIS2_PLACEMENT_3D ( 'NONE', #6118, #3535, #2685 ) ;
#3945=VERTEX_POINT ( 'NONE', #2655 ) ;
#3955=ORIENTED_EDGE ( 'NONE', *, *, #8119, .T. ) ;
#3970=CONICAL_SURFACE ( 'NONE', #8015, 4.000000000000003553, 1.029744258676655200 ) ;
#3982=VECTOR ( 'NONE', #6774, 1000.000000000000000 ) ;
#3984=DIRECTION ( 'NONE',  ( -0.000000000000000000, -0.000000000000000000, 1.000000000000000000 ) ) ;
#3997=EDGE_LOOP ( 'NONE', ( #1428, #2383, #6877, #4731 ) ) ;
#3999=DIRECTION ( 'NONE',  ( 1.000000000000000000, 0.000000000000000000, -1.137729606058012035E-16 ) ) ;
#4000=AXIS2_PLACEMENT_3D ( 'NONE', #8569, #518, #5388 ) ;
#4024=AXIS2_PLACEMENT_3D ( 'NONE', #6523, #3292, #9773 ) ;
#4038=CARTESIAN_POINT ( 'NONE',  ( -23.17384457509314544, 150.5696653505793563, -7.749999999999996447 ) ) ;
#4057=CARTESIAN_POINT ( 'NONE',  ( -3.173844575093148990, 105.5289575273812233, 10.90000000000000036 ) ) ;
#4060=EDGE_LOOP ( 'NONE', ( #3772, #140 ) ) ;
#4061=ADVANCED_FACE ( 'NONE', ( #8637 ), #6783, .F. ) ;
#4063=DIRECTION ( 'NONE',  ( 0.000000000000000000, 0.000000000000000000, 1.000000000000000000 ) ) ;
#4064=CYLINDRICAL_SURFACE ( 'NONE', #9209, 4.024999999999997691 ) ;
#4070=ORIENTED_EDGE ( 'NONE', *, *, #9501, .F. ) ;
#4074=DIRECTION ( 'NONE',  ( -1.000000000000000000, -0.000000000000000000, -0.000000000000000000 ) ) ;
#4079=AXIS2_PLACEMENT_3D ( 'NONE', #6940, #5339, #1319 ) ;
#4090=CARTESIAN_POINT ( 'NONE',  ( -23.17384457509314899, 130.5696653505793847, -7.749999999999996447 ) ) ;
#4095=CIRCLE ( 'NONE', #38, 3.999999999999993339 ) ;
#4096=VERTEX_POINT ( 'NONE', #5985 ) ;
#4099=( NAMED_UNIT ( * ) PLANE_ANGLE_UNIT ( ) SI_UNIT ( $, .RADIAN. ) );
#4104=DIRECTION ( 'NONE',  ( 0.000000000000000000, 0.000000000000000000, 1.000000000000000000 ) ) ;
#4106=CARTESIAN_POINT ( 'NONE',  ( -23.17384457509314899, 150.5696653505793563, 10.90000000000000036 ) ) ;
#4113=CIRCLE ( 'NONE', #9188, 5.000000000000004441 ) ;
#4121=ADVANCED_FACE ( 'NONE', ( #5507 ), #4664, .F. ) ;
#4127=CARTESIAN_POINT ( 'NONE',  ( -3.173844575093148990, 130.5696653505793847, 10.90000000000000036 ) ) ;
#4135=EDGE_LOOP ( 'NONE', ( #5860, #2924, #7204, #1357 ) ) ;
#4136=VERTEX_POINT ( 'NONE', #4760 ) ;
#4141=CARTESIAN_POINT ( 'NONE',  ( -56.36957570605427037, 137.0132282531173473, 3.999999999999989786 ) ) ;
#4166=FACE_OUTER_BOUND ( 'NONE', #6437, .T. ) ;
#4182=DIRECTION ( 'NONE',  ( -1.000000000000000000, 0.000000000000000000, 1.734723475976805615E-16 ) ) ;
#4197=EDGE_LOOP ( 'NONE', ( #593, #6651, #537, #8794 ) ) ;
#4219=VERTEX_POINT ( 'NONE', #5609 ) ;
#4226=DIRECTION ( 'NONE',  ( 0.000000000000000000, 0.000000000000000000, 1.000000000000000000 ) ) ;
#4233=DIRECTION ( 'NONE',  ( -1.000000000000000000, 0.000000000000000000, 0.000000000000000000 ) ) ;
#4243=CARTESIAN_POINT ( 'NONE',  ( -47.94539818030330025, 137.0132282531173473, -3.999999999999991562 ) ) ;
#4254=LINE ( 'NONE', #6689, #5871 ) ;
#4255=( NAMED_UNIT ( * ) SI_UNIT ( $, .STERADIAN. ) SOLID_ANGLE_UNIT ( ) );
#4266=ORIENTED_EDGE ( 'NONE', *, *, #1427, .T. ) ;
#4274=CARTESIAN_POINT ( 'NONE',  ( -47.94539818030330025, 150.5696653505793563, 0.000000000000000000 ) ) ;
#4276=CIRCLE ( 'NONE', #6790, 5.000000000000004441 ) ;
#4281=DIRECTION ( 'NONE',  ( 1.000000000000000000, 0.000000000000000000, 0.000000000000000000 ) ) ;
#4288=ORIENTED_EDGE ( 'NONE', *, *, #3204, .T. ) ;
#4289=AXIS2_PLACEMENT_3D ( 'NONE', #2283, #1000, #4233 ) ;
#4296=AXIS2_PLACEMENT_3D ( 'NONE', #5004, #8247, #4951 ) ;
#4309=EDGE_CURVE ( 'NONE', #4219, #4136, #8379, .T. ) ;
#4310=EDGE_CURVE ( 'NONE', #3419, #8839, #6003, .T. ) ;
#4314=AXIS2_PLACEMENT_3D ( 'NONE', #9610, #2338, #4762 ) ;
#4316=CYLINDRICAL_SURFACE ( 'NONE', #2922, 3.999999999999989786 ) ;
#4343=VERTEX_POINT ( 'NONE', #2695 ) ;
#4357=EDGE_CURVE ( 'NONE', #4343, #3877, #3470, .T. ) ;
#4371=FACE_OUTER_BOUND ( 'NONE', #4135, .T. ) ;
#4376=FACE_OUTER_BOUND ( 'NONE', #2798, .T. ) ;
#4381=CARTESIAN_POINT ( 'NONE',  ( -36.36957570605426326, 137.0132282531173473, 0.000000000000000000 ) ) ;
#4417=DIRECTION ( 'NONE',  ( 8.659560562357336419E-17, 0.7071067811863512853, -0.7071067811867437491 ) ) ;
#4420=CARTESIAN_POINT ( 'NONE',  ( -3.173844575093148990, 105.5289575273812233, 10.90000000000000036 ) ) ;
#4423=DIRECTION ( 'NONE',  ( -0.000000000000000000, 1.000000000000000000, -0.000000000000000000 ) ) ;
#4425=EDGE_CURVE ( 'NONE', #5689, #2102, #7627, .T. ) ;
#4429=CARTESIAN_POINT ( 'NONE',  ( -3.173844575093148990, 105.5289575273812233, -7.750000000000000000 ) ) ;
#4444=EDGE_CURVE ( 'NONE', #5509, #9513, #8883, .T. ) ;
#4452=CARTESIAN_POINT ( 'NONE',  ( -16.26850689640809833, 140.5696653505793563, 10.90000000000000036 ) ) ;
#4484=CARTESIAN_POINT ( 'NONE',  ( -27.85255513972543895, 64.37996872128307757, 7.750000000000002665 ) ) ;
#4507=FACE_OUTER_BOUND ( 'NONE', #9738, .T. ) ;
#4514=EDGE_LOOP ( 'NONE', ( #3696, #10054, #9519, #7299 ) ) ;
#4519=DIRECTION ( 'NONE',  ( 0.000000000000000000, 0.000000000000000000, 1.000000000000000000 ) ) ;
#4520=AXIS2_PLACEMENT_3D ( 'NONE', #9150, #3431, #1890 ) ;
#4524=DIRECTION ( 'NONE',  ( -0.000000000000000000, 1.000000000000000000, -0.000000000000000000 ) ) ;
#4532=CARTESIAN_POINT ( 'NONE',  ( -39.94539818030332157, 129.0132282531173757, 3.999999999999988898 ) ) ;
#4553=ORIENTED_EDGE ( 'NONE', *, *, #4310, .F. ) ;
#4554=CARTESIAN_POINT ( 'NONE',  ( -56.36957570605427037, 137.0132282531173473, 0.000000000000000000 ) ) ;
#4579=DIRECTION ( 'NONE',  ( -1.000000000000000000, 0.000000000000000000, 0.000000000000000000 ) ) ;
#4601=AXIS2_PLACEMENT_3D ( 'NONE', #8586, #5983, #5928 ) ;
#4603=FACE_BOUND ( 'NONE', #8083, .T. ) ;
#4620=CARTESIAN_POINT ( 'NONE',  ( -47.94539818030330025, 90.52895752738122326, -3.999999999999993339 ) ) ;
#4632=FACE_BOUND ( 'NONE', #4858, .T. ) ;
#4644=FACE_OUTER_BOUND ( 'NONE', #854, .T. ) ;
#4645=ORIENTED_EDGE ( 'NONE', *, *, #5347, .T. ) ;
#4650=CARTESIAN_POINT ( 'NONE',  ( -24.31850689640809549, 140.5696653505793563, 10.90000000000000036 ) ) ;
#4657=EDGE_LOOP ( 'NONE', ( #4553, #3084, #2950, #6461 ) ) ;
#4664=CYLINDRICAL_SURFACE ( 'NONE', #8768, 5.000000000000004441 ) ;
#4666=CARTESIAN_POINT ( 'NONE',  ( -20.29350689640809691, 140.5696653505793563, 7.750000000000001776 ) ) ;
#4671=VECTOR ( 'NONE', #1678, 1000.000000000000114 ) ;
#4698=ORIENTED_EDGE ( 'NONE', *, *, #8630, .T. ) ;
#4717=CIRCLE ( 'NONE', #154, 4.024999999999997691 ) ;
#4725=CARTESIAN_POINT ( 'NONE',  ( -47.94539818030330025, 150.5696653505793563, 0.000000000000000000 ) ) ;
#4727=CYLINDRICAL_SURFACE ( 'NONE', #5463, 3.999999999999989786 ) ;
#4731=ORIENTED_EDGE ( 'NONE', *, *, #6433, .F. ) ;
#4738=ORIENTED_EDGE ( 'NONE', *, *, #9049, .T. ) ;
#4760=CARTESIAN_POINT ( 'NONE',  ( -21.29350689640810046, 105.5289575273812233, 10.90000000000000036 ) ) ;
#4762=DIRECTION ( 'NONE',  ( 0.000000000000000000, 0.000000000000000000, 1.000000000000000000 ) ) ;
#4801=EDGE_CURVE ( 'NONE', #5649, #5184, #2468, .T. ) ;
#4808=PLANE ( 'NONE',  #5632 ) ;
#4813=ORIENTED_EDGE ( 'NONE', *, *, #9049, .F. ) ;
#4824=VERTEX_POINT ( 'NONE', #2683 ) ;
#4827=DIRECTION ( 'NONE',  ( -0.000000000000000000, 1.000000000000000000, -0.000000000000000000 ) ) ;
#4840=DIRECTION ( 'NONE',  ( 0.000000000000000000, 0.000000000000000000, -1.000000000000000000 ) ) ;
#4858=EDGE_LOOP ( 'NONE', ( #7747, #2374 ) ) ;
#4862=LINE ( 'NONE', #840, #8694 ) ;
#4899=DIRECTION ( 'NONE',  ( -1.000000000000000000, 0.000000000000000000, 0.000000000000000000 ) ) ;
#4902=DIRECTION ( 'NONE',  ( -0.000000000000000000, 1.000000000000000000, -0.000000000000000000 ) ) ;
#4916=EDGE_CURVE ( 'NONE', #2551, #3355, #6709, .T. ) ;
#4918=CARTESIAN_POINT ( 'NONE',  ( -56.36957570605427037, 137.0132282531173473, 0.000000000000000000 ) ) ;
#4928=AXIS2_PLACEMENT_3D ( 'NONE', #4725, #1445, #7913 ) ;
#4930=EDGE_CURVE ( 'NONE', #8839, #3419, #6359, .T. ) ;
#4939=DIRECTION ( 'NONE',  ( 1.000000000000000000, 0.000000000000000000, -1.734723475976805615E-16 ) ) ;
#4951=DIRECTION ( 'NONE',  ( -1.000000000000000000, 0.000000000000000000, 0.000000000000000000 ) ) ;
#4996=CARTESIAN_POINT ( 'NONE',  ( -23.17384457509314899, 130.5696653505793847, 10.90000000000000036 ) ) ;
#4999=VECTOR ( 'NONE', #236, 1000.000000000000000 ) ;
#5004=CARTESIAN_POINT ( 'NONE',  ( -20.29350689640809691, 140.5696653505793563, -7.749999999999996447 ) ) ;
#5015=CARTESIAN_POINT ( 'NONE',  ( -16.26850689640809833, 140.5696653505793563, 7.750000000000000888 ) ) ;
#5022=DIRECTION ( 'NONE',  ( 1.000000000000000000, 0.000000000000000000, -0.000000000000000000 ) ) ;
#5034=LINE ( 'NONE', #4141, #7494 ) ;
#5048=VECTOR ( 'NONE', #8042, 1000.000000000000000 ) ;
#5070=EDGE_CURVE ( 'NONE', #2663, #84, #5340, .T. ) ;
#5075=DIRECTION ( 'NONE',  ( 0.000000000000000000, 0.000000000000000000, 1.000000000000000000 ) ) ;
#5076=DIRECTION ( 'NONE',  ( 0.000000000000000000, 0.000000000000000000, 1.000000000000000000 ) ) ;
#5095=ORIENTED_EDGE ( 'NONE', *, *, #6587, .T. ) ;
#5118=DIRECTION ( 'NONE',  ( -1.000000000000000000, -0.000000000000000000, -0.000000000000000000 ) ) ;
#5151=PLANE ( 'NONE',  #3748 ) ;
#5154=PLANE ( 'NONE',  #2442 ) ;
#5169=FACE_OUTER_BOUND ( 'NONE', #4197, .T. ) ;
#5171=ORIENTED_EDGE ( 'NONE', *, *, #6432, .F. ) ;
#5180=DIRECTION ( 'NONE',  ( 0.000000000000000000, 0.000000000000000000, 1.000000000000000000 ) ) ;
#5184=VERTEX_POINT ( 'NONE', #3412 ) ;
#5197=VERTEX_POINT ( 'NONE', #6647 ) ;
#5206=EDGE_CURVE ( 'NONE', #382, #7686, #7521, .T. ) ;
#5226=VERTEX_POINT ( 'NONE', #5944 ) ;
#5229=AXIS2_PLACEMENT_3D ( 'NONE', #4420, #2775, #10205 ) ;
#5242=ORIENTED_EDGE ( 'NONE', *, *, #9228, .F. ) ;
#5248=EDGE_LOOP ( 'NONE', ( #7275, #1004, #7975, #7562, #3482 ) ) ;
#5257=DIRECTION ( 'NONE',  ( -0.000000000000000000, -0.000000000000000000, -1.000000000000000000 ) ) ;
#5283=CYLINDRICAL_SURFACE ( 'NONE', #2269, 5.000000000000004441 ) ;
#5299=CIRCLE ( 'NONE', #8351, 4.000000000000003553 ) ;
#5300=EDGE_LOOP ( 'NONE', ( #6020, #6, #7229, #2864 ) ) ;
#5301=ORIENTED_EDGE ( 'NONE', *, *, #1453, .F. ) ;
#5339=DIRECTION ( 'NONE',  ( 0.000000000000000000, -0.000000000000000000, 1.000000000000000000 ) ) ;
#5340=CIRCLE ( 'NONE', #769, 4.024999999999997691 ) ;
#5343=CIRCLE ( 'NONE', #1458, 4.000000000000003553 ) ;
#5347=EDGE_CURVE ( 'NONE', #7785, #8880, #9767, .T. ) ;
#5383=AXIS2_PLACEMENT_3D ( 'NONE', #6403, #2375, #5607 ) ;
#5387=ORIENTED_EDGE ( 'NONE', *, *, #8448, .T. ) ;
#5388=DIRECTION ( 'NONE',  ( 1.000000000000000000, 0.000000000000000000, 0.000000000000000000 ) ) ;
#5407=ORIENTED_EDGE ( 'NONE', *, *, #8630, .F. ) ;
#5411=EDGE_CURVE ( 'NONE', #5226, #2102, #1289, .T. ) ;
#5432=ADVANCED_BREP_SHAPE_REPRESENTATION ( '', ( #9943, #4601 ), #409 ) ;
#5435=DIRECTION ( 'NONE',  ( -0.7071067811863512853, 8.659560562357336419E-17, -0.7071067811867437491 ) ) ;
#5442=CARTESIAN_POINT ( 'NONE',  ( -56.34457570605425758, 137.0132282531173473, -3.999999999999976019 ) ) ;
#5460=DIRECTION ( 'NONE',  ( 1.137729606058012035E-16, 0.000000000000000000, 1.000000000000000000 ) ) ;
#5463=AXIS2_PLACEMENT_3D ( 'NONE', #9566, #9669, #12 ) ;
#5475=DIRECTION ( 'NONE',  ( 1.000000000000000000, 0.000000000000000000, 0.000000000000000000 ) ) ;
#5499=EDGE_CURVE ( 'NONE', #7087, #10167, #2822, .T. ) ;
#5507=FACE_OUTER_BOUND ( 'NONE', #3093, .T. ) ;
#5509=VERTEX_POINT ( 'NONE', #960 ) ;
#5518=CARTESIAN_POINT ( 'NONE',  ( -56.36957570605427748, 150.5696653505793563, 10.90000000000000036 ) ) ;
#5541=SHAPE_DEFINITION_REPRESENTATION ( #7796, #286 ) ;
#5555=CIRCLE ( 'NONE', #5383, 20.00000000000000000 ) ;
#5558=LINE ( 'NONE', #9699, #8578 ) ;
#5573=DIRECTION ( 'NONE',  ( -1.000000000000000000, -0.000000000000000000, -0.000000000000000000 ) ) ;
#5607=DIRECTION ( 'NONE',  ( 1.000000000000000000, -1.387778780781445676E-15, -1.301042606982605321E-16 ) ) ;
#5609=CARTESIAN_POINT ( 'NONE',  ( -11.29350689640809158, 105.5289575273812233, 10.90000000000000036 ) ) ;
#5619=FACE_OUTER_BOUND ( 'NONE', #684, .T. ) ;
#5626=AXIS2_PLACEMENT_3D ( 'NONE', #4996, #4840, #8079 ) ;
#5632=AXIS2_PLACEMENT_3D ( 'NONE', #3929, #7207, #1435 ) ;
#5649=VERTEX_POINT ( 'NONE', #1372 ) ;
#5686=CYLINDRICAL_SURFACE ( 'NONE', #5626, 20.00000000000000000 ) ;
#5689=VERTEX_POINT ( 'NONE', #281 ) ;
#5690=CARTESIAN_POINT ( 'NONE',  ( -16.26850689640809833, 140.5696653505793563, 10.90000000000000036 ) ) ;
#5695=CARTESIAN_POINT ( 'NONE',  ( -36.36957570605426326, 137.0132282531173473, -4.000000000000003553 ) ) ;
#5708=CARTESIAN_POINT ( 'NONE',  ( -3.173844575093148990, 90.52895752738122326, 10.90000000000000036 ) ) ;
#5717=VECTOR ( 'NONE', #3663, 1000.000000000000000 ) ;
#5760=CARTESIAN_POINT ( 'NONE',  ( -16.29350689640809691, 105.5289575273812233, -7.749999999999996447 ) ) ;
#5795=ORIENTED_EDGE ( 'NONE', *, *, #6655, .T. ) ;
#5829=AXIS2_PLACEMENT_3D ( 'NONE', #7362, #2536, #8264 ) ;
#5836=ORIENTED_EDGE ( 'NONE', *, *, #1336, .T. ) ;
#5845=DIRECTION ( 'NONE',  ( 0.000000000000000000, -0.000000000000000000, 1.000000000000000000 ) ) ;
#5853=LINE ( 'NONE', #6009, #1977 ) ;
#5860=ORIENTED_EDGE ( 'NONE', *, *, #1427, .F. ) ;
#5871=VECTOR ( 'NONE', #9991, 1000.000000000000000 ) ;
#5878=ADVANCED_FACE ( 'NONE', ( #3271 ), #8942, .F. ) ;
#5879=DIRECTION ( 'NONE',  ( 0.000000000000000000, 0.000000000000000000, 1.000000000000000000 ) ) ;
#5887=ORIENTED_EDGE ( 'NONE', *, *, #9037, .F. ) ;
#5890=ORIENTED_EDGE ( 'NONE', *, *, #9890, .T. ) ;
#5896=CIRCLE ( 'NONE', #10474, 5.000000000000004441 ) ;
#5903=ORIENTED_EDGE ( 'NONE', *, *, #934, .F. ) ;
#5911=VECTOR ( 'NONE', #8572, 1000.000000000000000 ) ;
#5918=ADVANCED_FACE ( 'NONE', ( #8139 ), #7405, .F. ) ;
#5928=DIRECTION ( 'NONE',  ( 1.000000000000000000, 0.000000000000000000, 0.000000000000000000 ) ) ;
#5931=CARTESIAN_POINT ( 'NONE',  ( -21.29350689640810046, 105.5289575273812233, -7.749999999999995559 ) ) ;
#5935=ORIENTED_EDGE ( 'NONE', *, *, #2172, .T. ) ;
#5944=CARTESIAN_POINT ( 'NONE',  ( -27.85255513972543895, 90.52895752738122326, 7.750000000000002665 ) ) ;
#5945=AXIS2_PLACEMENT_3D ( 'NONE', #7359, #9053, #6668 ) ;
#5950=ORIENTED_EDGE ( 'NONE', *, *, #4425, .F. ) ;
#5951=PLANE ( 'NONE',  #5229 ) ;
#5955=( LENGTH_UNIT ( ) NAMED_UNIT ( * ) SI_UNIT ( .MILLI., .METRE. ) );
#5957=FACE_OUTER_BOUND ( 'NONE', #3555, .T. ) ;
#5966=EDGE_CURVE ( 'NONE', #8839, #6132, #1836, .T. ) ;
#5983=DIRECTION ( 'NONE',  ( 0.000000000000000000, 0.000000000000000000, 1.000000000000000000 ) ) ;
#5985=CARTESIAN_POINT ( 'NONE',  ( -3.173844575093148990, 90.52895752738122326, 7.750000000000000000 ) ) ;
#5991=DIRECTION ( 'NONE',  ( -0.000000000000000000, 1.000000000000000000, -0.000000000000000000 ) ) ;
#6002=CARTESIAN_POINT ( 'NONE',  ( -56.36957570605427037, 137.0132282531173473, 0.000000000000000000 ) ) ;
#6003=CIRCLE ( 'NONE', #2624, 3.999999999999976019 ) ;
#6009=CARTESIAN_POINT ( 'NONE',  ( -47.94539818030330025, 150.5696653505793563, 3.999999999999993339 ) ) ;
#6012=LINE ( 'NONE', #4429, #2231 ) ;
#6020=ORIENTED_EDGE ( 'NONE', *, *, #6202, .F. ) ;
#6032=DIRECTION ( 'NONE',  ( -0.000000000000000000, -0.000000000000000000, -1.000000000000000000 ) ) ;
#6034=AXIS2_PLACEMENT_3D ( 'NONE', #2086, #3045, #4579 ) ;
#6050=CARTESIAN_POINT ( 'NONE',  ( -55.94539818030328604, 145.0132282531173189, 3.999999999999990230 ) ) ;
#6055=ADVANCED_FACE ( 'NONE', ( #6121 ), #2838, .F. ) ;
#6059=LINE ( 'NONE', #8342, #1906 ) ;
#6070=DIRECTION ( 'NONE',  ( -1.000000000000000000, 0.000000000000000000, -0.000000000000000000 ) ) ;
#6083=CARTESIAN_POINT ( 'NONE',  ( -36.36957570605426326, 137.0132282531173473, 4.000000000000003553 ) ) ;
#6091=DIRECTION ( 'NONE',  ( 0.000000000000000000, 0.000000000000000000, 1.000000000000000000 ) ) ;
#6097=ORIENTED_EDGE ( 'NONE', *, *, #5499, .T. ) ;
#6100=FACE_BOUND ( 'NONE', #1684, .T. ) ;
#6106=CARTESIAN_POINT ( 'NONE',  ( -16.29350689640809691, 105.5289575273812233, -10.90000000000000036 ) ) ;
#6110=ADVANCED_FACE ( 'NONE', ( #5169 ), #8354, .F. ) ;
#6118=CARTESIAN_POINT ( 'NONE',  ( -20.29350689640809691, 140.5696653505793563, 10.90000000000000036 ) ) ;
#6121=FACE_OUTER_BOUND ( 'NONE', #1566, .T. ) ;
#6132=VERTEX_POINT ( 'NONE', #8408 ) ;
#6143=DIRECTION ( 'NONE',  ( -1.000000000000000000, 0.000000000000000000, 0.000000000000000000 ) ) ;
#6155=FACE_BOUND ( 'NONE', #8431, .T. ) ;
#6162=CYLINDRICAL_SURFACE ( 'NONE', #9161, 5.000000000000004441 ) ;
#6190=DIRECTION ( 'NONE',  ( -1.000000000000000000, -0.000000000000000000, -0.000000000000000000 ) ) ;
#6202=EDGE_CURVE ( 'NONE', #7686, #5509, #9469, .T. ) ;
#6204=ORIENTED_EDGE ( 'NONE', *, *, #6493, .T. ) ;
#6231=VERTEX_POINT ( 'NONE', #614 ) ;
#6235=VERTEX_POINT ( 'NONE', #2258 ) ;
#6245=VERTEX_POINT ( 'NONE', #1519 ) ;
#6268=CARTESIAN_POINT ( 'NONE',  ( -39.94539818030332157, 145.0132282531173189, 3.999999999999991562 ) ) ;
#6285=CONICAL_SURFACE ( 'NONE', #7642, 4.025000000000000355, 0.7853981633977258348 ) ;
#6289=CARTESIAN_POINT ( 'NONE',  ( -56.36957570605427748, 150.5696653505793563, -10.90000000000000036 ) ) ;
#6303=ORIENTED_EDGE ( 'NONE', *, *, #8186, .T. ) ;
#6311=EDGE_CURVE ( 'NONE', #6817, #4824, #9705, .T. ) ;
#6331=CARTESIAN_POINT ( 'NONE',  ( -47.94539818030330025, 137.0132282531173473, 3.999999999999991562 ) ) ;
#6346=CARTESIAN_POINT ( 'NONE',  ( -16.29350689640809691, 105.5289575273812233, -25.04213562373096380 ) ) ;
#6358=DIRECTION ( 'NONE',  ( 1.000000000000000000, 0.000000000000000000, 0.000000000000000000 ) ) ;
#6359=CIRCLE ( 'NONE', #277, 3.999999999999976019 ) ;
#6360=CYLINDRICAL_SURFACE ( 'NONE', #4314, 3.999999999999989786 ) ;
#6363=VECTOR ( 'NONE', #343, 1000.000000000000000 ) ;
#6369=LINE ( 'NONE', #5518, #10277 ) ;
#6390=VERTEX_POINT ( 'NONE', #1771 ) ;
#6402=ORIENTED_EDGE ( 'NONE', *, *, #615, .T. ) ;
#6403=CARTESIAN_POINT ( 'NONE',  ( -23.17384457509314899, 130.5696653505793847, 7.750000000000001776 ) ) ;
#6417=DIRECTION ( 'NONE',  ( 3.081165567444019513E-16, -1.000000000000000000, 0.000000000000000000 ) ) ;
#6423=ADVANCED_FACE ( 'NONE', ( #2458 ), #5686, .T. ) ;
#6428=( BOUNDED_CURVE ( )  B_SPLINE_CURVE ( 3, ( #2198, #7084, #4532, #6331 ),
 .UNSPECIFIED., .F., .T. ) 
 B_SPLINE_CURVE_WITH_KNOTS ( ( 4, 4 ),
 ( 1.570796326794896558, 4.712388980384689674 ),
 .UNSPECIFIED. ) 
 CURVE ( )  GEOMETRIC_REPRESENTATION_ITEM ( )  RATIONAL_B_SPLINE_CURVE ( ( 1.000000000000000000, 0.3333333333333333703, 0.3333333333333333703, 1.000000000000000000 ) ) 
 REPRESENTATION_ITEM ( '' )  );
#6432=EDGE_CURVE ( 'NONE', #5197, #6817, #821, .T. ) ;
#6433=EDGE_CURVE ( 'NONE', #4824, #8741, #8930, .T. ) ;
#6437=EDGE_LOOP ( 'NONE', ( #3712, #9205, #122, #3293 ) ) ;
#6448=ORIENTED_EDGE ( 'NONE', *, *, #1243, .F. ) ;
#6455=DIRECTION ( 'NONE',  ( -0.000000000000000000, 1.000000000000000000, -0.000000000000000000 ) ) ;
#6456=FACE_BOUND ( 'NONE', #9284, .T. ) ;
#6461=ORIENTED_EDGE ( 'NONE', *, *, #5966, .F. ) ;
#6466=DIRECTION ( 'NONE',  ( -0.000000000000000000, 1.000000000000000000, -0.000000000000000000 ) ) ;
#6493=EDGE_CURVE ( 'NONE', #5509, #3393, #3522, .T. ) ;
#6510=CARTESIAN_POINT ( 'NONE',  ( -23.17384457509314899, 150.5696653505793563, -10.90000000000000036 ) ) ;
#6523=CARTESIAN_POINT ( 'NONE',  ( -47.94539818030330025, 90.52895752738122326, 0.000000000000000000 ) ) ;
#6529=EDGE_CURVE ( 'NONE', #9834, #10419, #4276, .T. ) ;
#6540=DIRECTION ( 'NONE',  ( 1.000000000000000000, 0.000000000000000000, 0.000000000000000000 ) ) ;
#6542=DIRECTION ( 'NONE',  ( 1.000000000000000000, 0.000000000000000000, 0.000000000000000000 ) ) ;
#6550=CARTESIAN_POINT ( 'NONE',  ( -3.173844575093148990, 90.52895752738122326, 10.90000000000000036 ) ) ;
#6554=CARTESIAN_POINT ( 'NONE',  ( -56.36957570605427037, 137.0132282531173473, 4.025000000000000355 ) ) ;
#6556=EDGE_CURVE ( 'NONE', #84, #3945, #6059, .T. ) ;
#6557=ADVANCED_FACE ( 'NONE', ( #4371 ), #4316, .F. ) ;
#6559=AXIS2_PLACEMENT_3D ( 'NONE', #10414, #1457, #3999 ) ;
#6586=ORIENTED_EDGE ( 'NONE', *, *, #3348, .F. ) ;
#6587=EDGE_CURVE ( 'NONE', #4136, #4219, #4113, .T. ) ;
#6613=DIRECTION ( 'NONE',  ( -9.101836848464095537E-17, -0.000000000000000000, -1.000000000000000000 ) ) ;
#6615=ADVANCED_FACE ( 'NONE', ( #7177 ), #6162, .F. ) ;
#6635=AXIS2_PLACEMENT_3D ( 'NONE', #1112, #6730, #9333 ) ;
#6636=ORIENTED_EDGE ( 'NONE', *, *, #3733, .F. ) ;
#6647=CARTESIAN_POINT ( 'NONE',  ( -3.173844575093148990, 90.52895752738122326, 10.90000000000000036 ) ) ;
#6651=ORIENTED_EDGE ( 'NONE', *, *, #3008, .T. ) ;
#6655=EDGE_CURVE ( 'NONE', #5226, #10069, #7921, .T. ) ;
#6668=DIRECTION ( 'NONE',  ( 1.000000000000000000, 0.000000000000000000, -0.000000000000000000 ) ) ;
#6670=LINE ( 'NONE', #5708, #9557 ) ;
#6680=VECTOR ( 'NONE', #7365, 1000.000000000000000 ) ;
#6689=CARTESIAN_POINT ( 'NONE',  ( -23.17384457509314899, 150.5696653505793563, 10.90000000000000036 ) ) ;
#6693=DIRECTION ( 'NONE',  ( 0.000000000000000000, -1.000000000000000000, 0.000000000000000000 ) ) ;
#6709=LINE ( 'NONE', #254, #2126 ) ;
#6718=ORIENTED_EDGE ( 'NONE', *, *, #805, .F. ) ;
#6730=DIRECTION ( 'NONE',  ( -1.000000000000000000, -0.000000000000000000, -0.000000000000000000 ) ) ;
#6774=DIRECTION ( 'NONE',  ( -0.000000000000000000, -0.000000000000000000, 1.000000000000000000 ) ) ;
#6783=PLANE ( 'NONE',  #2331 ) ;
#6784=VECTOR ( 'NONE', #2904, 1000.000000000000114 ) ;
#6788=FACE_OUTER_BOUND ( 'NONE', #10149, .T. ) ;
#6790=AXIS2_PLACEMENT_3D ( 'NONE', #6106, #2827, #9350 ) ;
#6793=MECHANICAL_DESIGN_GEOMETRIC_PRESENTATION_REPRESENTATION('',(#866),#2388);
#6794=CARTESIAN_POINT ( 'NONE',  ( -47.94539818030330025, 137.0132282531173473, 3.999999999999991562 ) ) ;
#6809=DIRECTION ( 'NONE',  ( 0.000000000000000000, 0.000000000000000000, 1.000000000000000000 ) ) ;
#6817=VERTEX_POINT ( 'NONE', #8743 ) ;
#6831=ORIENTED_EDGE ( 'NONE', *, *, #240, .F. ) ;
#6840=DIRECTION ( 'NONE',  ( -1.000000000000000000, 0.000000000000000000, 0.000000000000000000 ) ) ;
#6852=CARTESIAN_POINT ( 'NONE',  ( -47.94539818030330025, 137.0132282531173473, -3.999999999999991562 ) ) ;
#6865=DIRECTION ( 'NONE',  ( -0.000000000000000000, 1.000000000000000000, -0.000000000000000000 ) ) ;
#6877=ORIENTED_EDGE ( 'NONE', *, *, #1053, .F. ) ;
#6887=EDGE_LOOP ( 'NONE', ( #2220, #2856 ) ) ;
#6888=ORIENTED_EDGE ( 'NONE', *, *, #9935, .F. ) ;
#6891=VECTOR ( 'NONE', #610, 1000.000000000000000 ) ;
#6898=ADVANCED_FACE ( 'NONE', ( #2532, #9702, #9917 ), #8259, .F. ) ;
#6924=FACE_OUTER_BOUND ( 'NONE', #2380, .T. ) ;
#6926=DIRECTION ( 'NONE',  ( 0.000000000000000000, 0.000000000000000000, 1.000000000000000000 ) ) ;
#6931=ORIENTED_EDGE ( 'NONE', *, *, #5070, .T. ) ;
#6936=ORIENTED_EDGE ( 'NONE', *, *, #4309, .T. ) ;
#6940=CARTESIAN_POINT ( 'NONE',  ( 0.000000000000000000, 0.000000000000000000, 10.90000000000000036 ) ) ;
#6944=DIRECTION ( 'NONE',  ( 0.000000000000000000, 1.000000000000000000, 0.000000000000000000 ) ) ;
#6954=ORIENTED_EDGE ( 'NONE', *, *, #10283, .T. ) ;
#6980=ORIENTED_EDGE ( 'NONE', *, *, #2473, .F. ) ;
#7000=ORIENTED_EDGE ( 'NONE', *, *, #6655, .F. ) ;
#7005=DIRECTION ( 'NONE',  ( 0.000000000000000000, 0.000000000000000000, 1.000000000000000000 ) ) ;
#7009=ORIENTED_EDGE ( 'NONE', *, *, #677, .T. ) ;
#7016=VECTOR ( 'NONE', #6865, 1000.000000000000000 ) ;
#7019=CARTESIAN_POINT ( 'NONE',  ( -20.29350689640809691, 140.5696653505793563, -10.90000000000000036 ) ) ;
#7052=DIRECTION ( 'NONE',  ( 0.000000000000000000, -0.000000000000000000, 1.000000000000000000 ) ) ;
#7053=VECTOR ( 'NONE', #1842, 1000.000000000000000 ) ;
#7062=AXIS2_PLACEMENT_3D ( 'NONE', #4554, #9436, #7786 ) ;
#7076=CARTESIAN_POINT ( 'NONE',  ( -16.29350689640809691, 105.5289575273812233, 10.90000000000000036 ) ) ;
#7084=CARTESIAN_POINT ( 'NONE',  ( -39.94539818030332157, 129.0132282531173757, -3.999999999999991562 ) ) ;
#7087=VERTEX_POINT ( 'NONE', #3487 ) ;
#7109=CARTESIAN_POINT ( 'NONE',  ( -20.29350689640809691, 140.5696653505793563, 7.750000000000001776 ) ) ;
#7115=FACE_OUTER_BOUND ( 'NONE', #697, .T. ) ;
#7125=CARTESIAN_POINT ( 'NONE',  ( -39.94539818030332157, 145.0132282531173189, -3.999999999999988898 ) ) ;
#7128=DIRECTION ( 'NONE',  ( 0.000000000000000000, 0.000000000000000000, -1.000000000000000000 ) ) ;
#7137=AXIS2_PLACEMENT_3D ( 'NONE', #729, #8628, #9595 ) ;
#7142=ORIENTED_EDGE ( 'NONE', *, *, #5499, .F. ) ;
#7148=CARTESIAN_POINT ( 'NONE',  ( -47.94539818030330025, 150.5696653505793563, 4.025000000000000355 ) ) ;
#7163=ORIENTED_EDGE ( 'NONE', *, *, #894, .T. ) ;
#7177=FACE_OUTER_BOUND ( 'NONE', #7378, .T. ) ;
#7193=ORIENTED_EDGE ( 'NONE', *, *, #8790, .T. ) ;
#7204=ORIENTED_EDGE ( 'NONE', *, *, #3761, .T. ) ;
#7207=DIRECTION ( 'NONE',  ( 1.000000000000000000, 3.081165567444019513E-16, -0.000000000000000000 ) ) ;
#7229=ORIENTED_EDGE ( 'NONE', *, *, #3597, .T. ) ;
#7231=AXIS2_PLACEMENT_3D ( 'NONE', #8086, #8246, #4063 ) ;
#7244=VECTOR ( 'NONE', #3984, 1000.000000000000000 ) ;
#7245=EDGE_LOOP ( 'NONE', ( #407, #8154, #807, #8615 ) ) ;
#7264=VECTOR ( 'NONE', #4827, 1000.000000000000000 ) ;
#7272=CARTESIAN_POINT ( 'NONE',  ( -47.94539818030330025, 137.0132282531173473, -3.999999999999991562 ) ) ;
#7275=ORIENTED_EDGE ( 'NONE', *, *, #6432, .T. ) ;
#7291=LINE ( 'NONE', #9736, #2345 ) ;
#7299=ORIENTED_EDGE ( 'NONE', *, *, #3761, .F. ) ;
#7300=VECTOR ( 'NONE', #1671, 1000.000000000000000 ) ;
#7302=CARTESIAN_POINT ( 'NONE',  ( -21.29350689640810046, 105.5289575273812233, 7.750000000000000888 ) ) ;
#7305=DIRECTION ( 'NONE',  ( 1.137729606058012035E-16, 0.000000000000000000, 1.000000000000000000 ) ) ;
#7319=LINE ( 'NONE', #63, #9450 ) ;
#7331=ORIENTED_EDGE ( 'NONE', *, *, #690, .F. ) ;
#7359=CARTESIAN_POINT ( 'NONE',  ( 0.000000000000000000, 0.000000000000000000, -10.90000000000000036 ) ) ;
#7361=DIRECTION ( 'NONE',  ( -0.000000000000000000, 1.000000000000000000, -0.000000000000000000 ) ) ;
#7362=CARTESIAN_POINT ( 'NONE',  ( -16.29350689640809691, 105.5289575273812233, 10.90000000000000036 ) ) ;
#7365=DIRECTION ( 'NONE',  ( 3.081165567444019513E-16, -1.000000000000000000, 0.000000000000000000 ) ) ;
#7376=DIRECTION ( 'NONE',  ( 9.101836848464095537E-17, 0.000000000000000000, 1.000000000000000000 ) ) ;
#7378=EDGE_LOOP ( 'NONE', ( #2557, #8291, #7923, #3129 ) ) ;
#7381=UNCERTAINTY_MEASURE_WITH_UNIT (LENGTH_MEASURE( 1.000000000000000082E-05 ), #5955, 'distance_accuracy_value', 'NONE');
#7388=CARTESIAN_POINT ( 'NONE',  ( -16.26850689640809833, 140.5696653505793563, 10.90000000000000036 ) ) ;
#7401=LINE ( 'NONE', #6550, #9904 ) ;
#7405=CYLINDRICAL_SURFACE ( 'NONE', #9356, 3.999999999999993339 ) ;
#7452=( NAMED_UNIT ( * ) PLANE_ANGLE_UNIT ( ) SI_UNIT ( $, .RADIAN. ) );
#7471=ORIENTED_EDGE ( 'NONE', *, *, #10283, .F. ) ;
#7488=ORIENTED_EDGE ( 'NONE', *, *, #4444, .F. ) ;
#7494=VECTOR ( 'NONE', #8220, 1000.000000000000000 ) ;
#7501=VECTOR ( 'NONE', #7743, 1000.000000000000000 ) ;
#7521=( BOUNDED_CURVE ( )  B_SPLINE_CURVE ( 3, ( #9996, #3683, #8442, #8340 ),
 .UNSPECIFIED., .F., .F. ) 
 B_SPLINE_CURVE_WITH_KNOTS ( ( 4, 4 ),
 ( 4.712388980384689674, 7.853981633974482790 ),
 .UNSPECIFIED. ) 
 CURVE ( )  GEOMETRIC_REPRESENTATION_ITEM ( )  RATIONAL_B_SPLINE_CURVE ( ( 1.000000000000000000, 0.3333333333333333703, 0.3333333333333333703, 1.000000000000000000 ) ) 
 REPRESENTATION_ITEM ( '' )  );
#7528=CIRCLE ( 'NONE', #2289, 4.024999999999997691 ) ;
#7529=CARTESIAN_POINT ( 'NONE',  ( -16.26850689640809833, 140.5696653505793563, -10.90000000000000036 ) ) ;
#7545=FACE_BOUND ( 'NONE', #10427, .T. ) ;
#7555=ADVANCED_FACE ( 'NONE', ( #3835 ), #4727, .F. ) ;
#7559=DIRECTION ( 'NONE',  ( 0.000000000000000000, 0.000000000000000000, 1.000000000000000000 ) ) ;
#7562=ORIENTED_EDGE ( 'NONE', *, *, #1902, .T. ) ;
#7585=AXIS2_PLACEMENT_3D ( 'NONE', #4918, #8161, #5879 ) ;
#7588=DIRECTION ( 'NONE',  ( -1.000000000000000000, 0.000000000000000000, 0.000000000000000000 ) ) ;
#7618=EDGE_CURVE ( 'NONE', #382, #7686, #3591, .T. ) ;
#7626=DIRECTION ( 'NONE',  ( 1.000000000000000000, 0.000000000000000000, 0.000000000000000000 ) ) ;
#7627=LINE ( 'NONE', #1210, #3982 ) ;
#7636=VECTOR ( 'NONE', #6190, 1000.000000000000000 ) ;
#7637=ORIENTED_EDGE ( 'NONE', *, *, #6493, .F. ) ;
#7642=AXIS2_PLACEMENT_3D ( 'NONE', #3728, #1126, #4519 ) ;
#7655=ORIENTED_EDGE ( 'NONE', *, *, #7706, .F. ) ;
#7664=CARTESIAN_POINT ( 'NONE',  ( -47.94539818030330025, 150.5696653505793563, 0.000000000000000000 ) ) ;
#7669=LINE ( 'NONE', #10058, #459 ) ;
#7678=CARTESIAN_POINT ( 'NONE',  ( -47.94539818030330025, 150.5446653505793790, 0.000000000000000000 ) ) ;
#7686=VERTEX_POINT ( 'NONE', #4243 ) ;
#7704=ORIENTED_EDGE ( 'NONE', *, *, #615, .F. ) ;
#7706=EDGE_CURVE ( 'NONE', #382, #8839, #5034, .T. ) ;
#7714=EDGE_LOOP ( 'NONE', ( #2060, #4813, #9775, #2263 ) ) ;
#7720=ORIENTED_EDGE ( 'NONE', *, *, #9362, .F. ) ;
#7732=FACE_BOUND ( 'NONE', #2407, .T. ) ;
#7733=ORIENTED_EDGE ( 'NONE', *, *, #1324, .T. ) ;
#7742=CARTESIAN_POINT ( 'NONE',  ( -47.94539818030330025, 90.52895752738122326, 0.000000000000000000 ) ) ;
#7743=DIRECTION ( 'NONE',  ( -1.000000000000000000, 0.000000000000000000, 1.137729606058012035E-16 ) ) ;
#7747=ORIENTED_EDGE ( 'NONE', *, *, #9228, .T. ) ;
#7783=LINE ( 'NONE', #10229, #7636 ) ;
#7785=VERTEX_POINT ( 'NONE', #7529 ) ;
#7786=DIRECTION ( 'NONE',  ( 0.000000000000000000, 0.000000000000000000, 1.000000000000000000 ) ) ;
#7790=CARTESIAN_POINT ( 'NONE',  ( 10.26554134690924691, 90.52895752738122326, 7.749999999999998224 ) ) ;
#7792=CARTESIAN_POINT ( 'NONE',  ( -3.173844575093148990, 105.5289575273812233, 10.90000000000000036 ) ) ;
#7793=CARTESIAN_POINT ( 'NONE',  ( -3.173844575093148990, 150.5696653505793563, 10.90000000000000036 ) ) ;
#7796=PRODUCT_DEFINITION_SHAPE ( 'NONE', 'NONE',  #8329 ) ;
#7813=ORIENTED_EDGE ( 'NONE', *, *, #4310, .T. ) ;
#7816=DIRECTION ( 'NONE',  ( -0.000000000000000000, -0.000000000000000000, 1.000000000000000000 ) ) ;
#7832=LINE ( 'NONE', #7148, #907 ) ;
#7881=ORIENTED_EDGE ( 'NONE', *, *, #7928, .T. ) ;
#7884=CARTESIAN_POINT ( 'NONE',  ( -56.36957570605425616, 90.52895752738122326, 10.90000000000000036 ) ) ;
#7889=CIRCLE ( 'NONE', #9414, 20.00000000000000000 ) ;
#7910=VERTEX_POINT ( 'NONE', #8375 ) ;
#7913=DIRECTION ( 'NONE',  ( 0.000000000000000000, 0.000000000000000000, 1.000000000000000000 ) ) ;
#7921=LINE ( 'NONE', #3899, #9170 ) ;
#7923=ORIENTED_EDGE ( 'NONE', *, *, #4357, .F. ) ;
#7928=EDGE_CURVE ( 'NONE', #4096, #5226, #331, .T. ) ;
#7950=DIRECTION ( 'NONE',  ( 1.000000000000000000, 0.000000000000000000, -2.154935995002246132E-16 ) ) ;
#7956=EDGE_CURVE ( 'NONE', #6390, #6245, #3102, .T. ) ;
#7975=ORIENTED_EDGE ( 'NONE', *, *, #805, .T. ) ;
#7977=CARTESIAN_POINT ( 'NONE',  ( -47.94539818030330025, 150.5696653505793563, -3.999999999999993339 ) ) ;
#7987=CYLINDRICAL_SURFACE ( 'NONE', #7137, 4.024999999999997691 ) ;
#8007=DIRECTION ( 'NONE',  ( 0.000000000000000000, 0.000000000000000000, 1.000000000000000000 ) ) ;
#8015=AXIS2_PLACEMENT_3D ( 'NONE', #4381, #3693, #6809 ) ;
#8018=PRODUCT_DEFINITION_FORMATION_WITH_SPECIFIED_SOURCE ( 'ANY', '', #2307, .NOT_KNOWN. ) ;
#8020=ADVANCED_FACE ( 'NONE', ( #6456, #692 ), #4808, .F. ) ;
#8042=DIRECTION ( 'NONE',  ( -0.000000000000000000, -0.000000000000000000, 1.000000000000000000 ) ) ;
#8079=DIRECTION ( 'NONE',  ( -1.000000000000000000, 0.000000000000000000, 0.000000000000000000 ) ) ;
#8083=EDGE_LOOP ( 'NONE', ( #9818, #1510 ) ) ;
#8086=CARTESIAN_POINT ( 'NONE',  ( -56.36957570605427037, 137.0132282531173473, 0.000000000000000000 ) ) ;
#8104=ADVANCED_FACE ( 'NONE', ( #7115 ), #3071, .F. ) ;
#8119=EDGE_CURVE ( 'NONE', #5197, #4096, #6670, .T. ) ;
#8126=CARTESIAN_POINT ( 'NONE',  ( -20.29350689640809691, 140.5696653505793563, 10.90000000000000036 ) ) ;
#8139=FACE_OUTER_BOUND ( 'NONE', #5300, .T. ) ;
#8154=ORIENTED_EDGE ( 'NONE', *, *, #4930, .F. ) ;
#8156=ORIENTED_EDGE ( 'NONE', *, *, #8258, .F. ) ;
#8161=DIRECTION ( 'NONE',  ( -1.000000000000000000, -0.000000000000000000, -0.000000000000000000 ) ) ;
#8186=EDGE_CURVE ( 'NONE', #3393, #6231, #68, .T. ) ;
#8200=ORIENTED_EDGE ( 'NONE', *, *, #6202, .T. ) ;
#8217=ADVANCED_FACE ( 'NONE', ( #2480 ), #3490, .F. ) ;
#8220=DIRECTION ( 'NONE',  ( -1.000000000000000000, -0.000000000000000000, -0.000000000000000000 ) ) ;
#8224=CIRCLE ( 'NONE', #4000, 5.000000000000004441 ) ;
#8243=CONICAL_SURFACE ( 'NONE', #7231, 4.025000000000000355, 0.7853981633977258348 ) ;
#8246=DIRECTION ( 'NONE',  ( -1.000000000000000000, -0.000000000000000000, -0.000000000000000000 ) ) ;
#8247=DIRECTION ( 'NONE',  ( -9.101836848464095537E-17, -0.000000000000000000, -1.000000000000000000 ) ) ;
#8252=VERTEX_POINT ( 'NONE', #6510 ) ;
#8258=EDGE_CURVE ( 'NONE', #8552, #1166, #4862, .T. ) ;
#8259=PLANE ( 'NONE',  #5945 ) ;
#8260=EDGE_CURVE ( 'NONE', #10246, #5184, #5299, .T. ) ;
#8263=CARTESIAN_POINT ( 'NONE',  ( -36.36957570605426326, 137.0132282531173473, 0.000000000000000000 ) ) ;
#8264=DIRECTION ( 'NONE',  ( 1.000000000000000000, 0.000000000000000000, 0.000000000000000000 ) ) ;
#8279=ORIENTED_EDGE ( 'NONE', *, *, #8402, .T. ) ;
#8291=ORIENTED_EDGE ( 'NONE', *, *, #868, .T. ) ;
#8319=CARTESIAN_POINT ( 'NONE',  ( -3.173844575093148990, 105.5289575273812233, 7.750000000000000000 ) ) ;
#8329=PRODUCT_DEFINITION ( 'UNKNOWN', '', #8018, #2612 ) ;
#8335=LINE ( 'NONE', #9131, #28 ) ;
#8340=CARTESIAN_POINT ( 'NONE',  ( -47.94539818030330025, 137.0132282531173473, -3.999999999999991562 ) ) ;
#8342=CARTESIAN_POINT ( 'NONE',  ( -24.31850689640809549, 140.5696653505793563, 10.90000000000000036 ) ) ;
#8351=AXIS2_PLACEMENT_3D ( 'NONE', #8263, #3338, #9758 ) ;
#8353=ORIENTED_EDGE ( 'NONE', *, *, #4930, .T. ) ;
#8354=CYLINDRICAL_SURFACE ( 'NONE', #1560, 3.999999999999993339 ) ;
#8367=LINE ( 'NONE', #950, #6680 ) ;
#8370=ORIENTED_EDGE ( 'NONE', *, *, #10155, .T. ) ;
#8375=CARTESIAN_POINT ( 'NONE',  ( -3.173844575093148990, 130.5696653505793847, -10.90000000000000036 ) ) ;
#8379=CIRCLE ( 'NONE', #5829, 5.000000000000004441 ) ;
#8386=DIRECTION ( 'NONE',  ( -1.000000000000000000, 0.000000000000000000, 9.101836848464095537E-17 ) ) ;
#8402=EDGE_CURVE ( 'NONE', #84, #2663, #10051, .T. ) ;
#8406=AXIS2_PLACEMENT_3D ( 'NONE', #8579, #6944, #7052 ) ;
#8408=CARTESIAN_POINT ( 'NONE',  ( -56.36957570605427037, 137.0132282531173473, 4.025000000000000355 ) ) ;
#8412=ORIENTED_EDGE ( 'NONE', *, *, #4916, .F. ) ;
#8423=ORIENTED_EDGE ( 'NONE', *, *, #1336, .F. ) ;
#8431=EDGE_LOOP ( 'NONE', ( #2151, #4288 ) ) ;
#8436=ADVANCED_FACE ( 'NONE', ( #2052 ), #5283, .F. ) ;
#8442=CARTESIAN_POINT ( 'NONE',  ( -55.94539818030328604, 129.0132282531173757, -3.999999999999990230 ) ) ;
#8443=EDGE_LOOP ( 'NONE', ( #8683, #8496, #10377, #62 ) ) ;
#8448=EDGE_CURVE ( 'NONE', #9513, #6231, #7832, .T. ) ;
#8453=FACE_OUTER_BOUND ( 'NONE', #3997, .T. ) ;
#8474=FACE_OUTER_BOUND ( 'NONE', #1852, .T. ) ;
#8496=ORIENTED_EDGE ( 'NONE', *, *, #1453, .T. ) ;
#8513=ORIENTED_EDGE ( 'NONE', *, *, #9890, .F. ) ;
#8519=DIRECTION ( 'NONE',  ( -0.000000000000000000, 0.000000000000000000, -1.000000000000000000 ) ) ;
#8533=ORIENTED_EDGE ( 'NONE', *, *, #7928, .F. ) ;
#8542=VECTOR ( 'NONE', #9787, 1000.000000000000000 ) ;
#8543=ORIENTED_EDGE ( 'NONE', *, *, #6529, .F. ) ;
#8552=VERTEX_POINT ( 'NONE', #8831 ) ;
#8564=VECTOR ( 'NONE', #4524, 1000.000000000000000 ) ;
#8569=CARTESIAN_POINT ( 'NONE',  ( -16.29350689640809691, 105.5289575273812233, -10.90000000000000036 ) ) ;
#8572=DIRECTION ( 'NONE',  ( -0.000000000000000000, -0.000000000000000000, -1.000000000000000000 ) ) ;
#8576=LINE ( 'NONE', #6083, #6784 ) ;
#8578=VECTOR ( 'NONE', #1536, 1000.000000000000000 ) ;
#8579=CARTESIAN_POINT ( 'NONE',  ( -56.36957570605426326, 90.52895752738122326, 10.90000000000000036 ) ) ;
#8581=ADVANCED_FACE ( 'NONE', ( #4166 ), #4064, .F. ) ;
#8584=ORIENTED_EDGE ( 'NONE', *, *, #4309, .F. ) ;
#8586=CARTESIAN_POINT ( 'NONE',  ( 0.000000000000000000, 0.000000000000000000, 0.000000000000000000 ) ) ;
#8615=ORIENTED_EDGE ( 'NONE', *, *, #1974, .T. ) ;
#8620=ORIENTED_EDGE ( 'NONE', *, *, #240, .T. ) ;
#8628=DIRECTION ( 'NONE',  ( -0.000000000000000000, -0.000000000000000000, -1.000000000000000000 ) ) ;
#8630=EDGE_CURVE ( 'NONE', #6245, #6390, #245, .T. ) ;
#8637=FACE_OUTER_BOUND ( 'NONE', #9426, .T. ) ;
#8642=EDGE_CURVE ( 'NONE', #2784, #1166, #7401, .T. ) ;
#8655=DIRECTION ( 'NONE',  ( -0.000000000000000000, -0.000000000000000000, 1.000000000000000000 ) ) ;
#8683=ORIENTED_EDGE ( 'NONE', *, *, #868, .F. ) ;
#8694=VECTOR ( 'NONE', #5022, 1000.000000000000000 ) ;
#8741=VERTEX_POINT ( 'NONE', #1989 ) ;
#8743=CARTESIAN_POINT ( 'NONE',  ( -3.173844575093148990, 130.5696653505793847, 10.90000000000000036 ) ) ;
#8748=FACE_OUTER_BOUND ( 'NONE', #1467, .T. ) ;
#8755=ORIENTED_EDGE ( 'NONE', *, *, #3131, .F. ) ;
#8768=AXIS2_PLACEMENT_3D ( 'NONE', #1588, #1436, #6358 ) ;
#8776=ADVANCED_FACE ( 'NONE', ( #5957 ), #3970, .F. ) ;
#8790=EDGE_CURVE ( 'NONE', #10069, #5689, #404, .T. ) ;
#8794=ORIENTED_EDGE ( 'NONE', *, *, #691, .F. ) ;
#8831=CARTESIAN_POINT ( 'NONE',  ( -56.36957570605425616, 90.52895752738122326, -10.90000000000000036 ) ) ;
#8839=VERTEX_POINT ( 'NONE', #2143 ) ;
#8855=CARTESIAN_POINT ( 'NONE',  ( -21.29350689640810046, 105.5289575273812233, -25.04213562373096380 ) ) ;
#8868=ORIENTED_EDGE ( 'NONE', *, *, #4425, .T. ) ;
#8880=VERTEX_POINT ( 'NONE', #9410 ) ;
#8883=CIRCLE ( 'NONE', #10249, 3.999999999999989786 ) ;
#8926=DIRECTION ( 'NONE',  ( -0.000000000000000000, 0.000000000000000000, -1.000000000000000000 ) ) ;
#8930=LINE ( 'NONE', #4106, #1717 ) ;
#8942=CYLINDRICAL_SURFACE ( 'NONE', #386, 3.999999999999993339 ) ;
#8948=DIRECTION ( 'NONE',  ( -0.000000000000000000, -0.000000000000000000, 1.000000000000000000 ) ) ;
#8978=EDGE_CURVE ( 'NONE', #2082, #1644, #9573, .T. ) ;
#8981=LINE ( 'NONE', #7388, #8542 ) ;
#8993=DIRECTION ( 'NONE',  ( -0.000000000000000000, 1.000000000000000000, -0.000000000000000000 ) ) ;
#8995=ORIENTED_EDGE ( 'NONE', *, *, #4801, .T. ) ;
#9001=ORIENTED_EDGE ( 'NONE', *, *, #3597, .F. ) ;
#9037=EDGE_CURVE ( 'NONE', #2663, #2288, #8981, .T. ) ;
#9049=EDGE_CURVE ( 'NONE', #1535, #8552, #1610, .T. ) ;
#9051=ORIENTED_EDGE ( 'NONE', *, *, #1324, .F. ) ;
#9053=DIRECTION ( 'NONE',  ( 0.000000000000000000, -0.000000000000000000, 1.000000000000000000 ) ) ;
#9069=ORIENTED_EDGE ( 'NONE', *, *, #6556, .T. ) ;
#9108=CARTESIAN_POINT ( 'NONE',  ( -47.94539818030330025, 150.5696653505793563, 0.000000000000000000 ) ) ;
#9117=ORIENTED_EDGE ( 'NONE', *, *, #1976, .T. ) ;
#9131=CARTESIAN_POINT ( 'NONE',  ( -56.36957570605427037, 137.0132282531173473, -3.999999999999989786 ) ) ;
#9141=ADVANCED_FACE ( 'NONE', ( #7545, #2918 ), #5154, .F. ) ;
#9150=CARTESIAN_POINT ( 'NONE',  ( -47.94539818030330025, 150.5696653505793563, 0.000000000000000000 ) ) ;
#9161=AXIS2_PLACEMENT_3D ( 'NONE', #1508, #8655, #10410 ) ;
#9170=VECTOR ( 'NONE', #7128, 1000.000000000000000 ) ;
#9182=ORIENTED_EDGE ( 'NONE', *, *, #1200, .T. ) ;
#9184=FACE_OUTER_BOUND ( 'NONE', #10040, .T. ) ;
#9188=AXIS2_PLACEMENT_3D ( 'NONE', #7076, #3041, #5475 ) ;
#9205=ORIENTED_EDGE ( 'NONE', *, *, #7956, .F. ) ;
#9209=AXIS2_PLACEMENT_3D ( 'NONE', #877, #1621, #4899 ) ;
#9223=CARTESIAN_POINT ( 'NONE',  ( -3.173844575093148990, 150.5696653505793563, 10.90000000000000036 ) ) ;
#9228=EDGE_CURVE ( 'NONE', #3945, #2288, #7528, .T. ) ;
#9230=ADVANCED_FACE ( 'NONE', ( #8748 ), #6360, .F. ) ;
#9233=DIRECTION ( 'NONE',  ( 0.000000000000000000, 0.000000000000000000, 1.000000000000000000 ) ) ;
#9264=CARTESIAN_POINT ( 'NONE',  ( -23.17384457509314899, 130.5696653505793847, -10.90000000000000036 ) ) ;
#9284=EDGE_LOOP ( 'NONE', ( #661, #2183 ) ) ;
#9300=DIRECTION ( 'NONE',  ( -1.000000000000000000, -0.000000000000000000, -0.000000000000000000 ) ) ;
#9314=EDGE_LOOP ( 'NONE', ( #5407, #9117, #5903, #6586 ) ) ;
#9325=CARTESIAN_POINT ( 'NONE',  ( -47.94539818030330025, 150.5446653505793790, 3.999999999999989786 ) ) ;
#9333=DIRECTION ( 'NONE',  ( 0.000000000000000000, 0.000000000000000000, 1.000000000000000000 ) ) ;
#9344=DIRECTION ( 'NONE',  ( -9.101836848464095537E-17, 0.000000000000000000, -1.000000000000000000 ) ) ;
#9350=DIRECTION ( 'NONE',  ( 1.000000000000000000, 0.000000000000000000, 0.000000000000000000 ) ) ;
#9356=AXIS2_PLACEMENT_3D ( 'NONE', #3323, #8993, #4226 ) ;
#9362=EDGE_CURVE ( 'NONE', #3355, #8552, #8367, .T. ) ;
#9370=ORIENTED_EDGE ( 'NONE', *, *, #894, .F. ) ;
#9397=CARTESIAN_POINT ( 'NONE',  ( -27.85255513972543895, 90.52895752738122326, -7.749999999999996447 ) ) ;
#9410=CARTESIAN_POINT ( 'NONE',  ( -24.31850689640809549, 140.5696653505793563, -10.90000000000000036 ) ) ;
#9414=AXIS2_PLACEMENT_3D ( 'NONE', #9264, #8519, #4281 ) ;
#9420=EDGE_LOOP ( 'NONE', ( #7488, #6204, #6303, #9571 ) ) ;
#9422=CARTESIAN_POINT ( 'NONE',  ( -36.36957570605426326, 137.0132282531173473, 0.000000000000000000 ) ) ;
#9426=EDGE_LOOP ( 'NONE', ( #7009, #571, #5171, #3955 ) ) ;
#9436=DIRECTION ( 'NONE',  ( -1.000000000000000000, -0.000000000000000000, -0.000000000000000000 ) ) ;
#9450=VECTOR ( 'NONE', #6466, 1000.000000000000000 ) ;
#9458=VECTOR ( 'NONE', #6143, 1000.000000000000000 ) ;
#9469=LINE ( 'NONE', #7977, #9873 ) ;
#9481=CARTESIAN_POINT ( 'NONE',  ( -47.94539818030330025, 150.5696653505793563, -4.025000000000000355 ) ) ;
#9501=EDGE_CURVE ( 'NONE', #5649, #10246, #8576, .T. ) ;
#9513=VERTEX_POINT ( 'NONE', #9325 ) ;
#9516=APPLICATION_CONTEXT ( 'automotive_design' ) ;
#9519=ORIENTED_EDGE ( 'NONE', *, *, #691, .T. ) ;
#9526=ORIENTED_EDGE ( 'NONE', *, *, #10155, .F. ) ;
#9549=DIRECTION ( 'NONE',  ( 1.137729606058012035E-16, 0.000000000000000000, 1.000000000000000000 ) ) ;
#9557=VECTOR ( 'NONE', #3437, 1000.000000000000000 ) ;
#9566=CARTESIAN_POINT ( 'NONE',  ( -56.36957570605427037, 137.0132282531173473, 0.000000000000000000 ) ) ;
#9569=ADVANCED_FACE ( 'NONE', ( #7732, #474, #2112 ), #3709, .T. ) ;
#9571=ORIENTED_EDGE ( 'NONE', *, *, #8448, .F. ) ;
#9573=CIRCLE ( 'NONE', #250, 5.000000000000004441 ) ;
#9575=EDGE_CURVE ( 'NONE', #5184, #7686, #7783, .T. ) ;
#9595=DIRECTION ( 'NONE',  ( -1.000000000000000000, 0.000000000000000000, 0.000000000000000000 ) ) ;
#9604=CARTESIAN_POINT ( 'NONE',  ( -20.29350689640809691, 140.5696653505793563, -10.90000000000000036 ) ) ;
#9606=AXIS2_PLACEMENT_3D ( 'NONE', #4090, #7376, #808 ) ;
#9610=CARTESIAN_POINT ( 'NONE',  ( -56.36957570605427037, 137.0132282531173473, 0.000000000000000000 ) ) ;
#9626=AXIS2_PLACEMENT_3D ( 'NONE', #1391, #5573, #8007 ) ;
#9640=VECTOR ( 'NONE', #8948, 1000.000000000000000 ) ;
#9641=ADVANCED_FACE ( 'NONE', ( #3215 ), #7987, .F. ) ;
#9651=CIRCLE ( 'NONE', #502, 5.000000000000004441 ) ;
#9652=ORIENTED_EDGE ( 'NONE', *, *, #5411, .T. ) ;
#9669=DIRECTION ( 'NONE',  ( -1.000000000000000000, -0.000000000000000000, -0.000000000000000000 ) ) ;
#9672=CARTESIAN_POINT ( 'NONE',  ( -47.94539818030330025, 150.5696653505793563, -3.999999999999993339 ) ) ;
#9677=FACE_OUTER_BOUND ( 'NONE', #2202, .T. ) ;
#9699=CARTESIAN_POINT ( 'NONE',  ( -56.36957570605427037, 137.0132282531173473, 3.999999999999989786 ) ) ;
#9702=FACE_OUTER_BOUND ( 'NONE', #3196, .T. ) ;
#9705=CIRCLE ( 'NONE', #26, 20.00000000000000000 ) ;
#9729=CARTESIAN_POINT ( 'NONE',  ( -56.36957570605425616, 90.52895752738122326, 10.90000000000000036 ) ) ;
#9736=CARTESIAN_POINT ( 'NONE',  ( -56.36957570605427037, 137.0132282531173473, -4.025000000000000355 ) ) ;
#9738=EDGE_LOOP ( 'NONE', ( #9792, #10273, #1755 ) ) ;
#9758=DIRECTION ( 'NONE',  ( 0.000000000000000000, 0.000000000000000000, 1.000000000000000000 ) ) ;
#9767=CIRCLE ( 'NONE', #3492, 4.024999999999997691 ) ;
#9773=DIRECTION ( 'NONE',  ( 0.000000000000000000, 0.000000000000000000, 1.000000000000000000 ) ) ;
#9775=ORIENTED_EDGE ( 'NONE', *, *, #1902, .F. ) ;
#9785=DIRECTION ( 'NONE',  ( -1.000000000000000000, -0.000000000000000000, -0.000000000000000000 ) ) ;
#9787=DIRECTION ( 'NONE',  ( -0.000000000000000000, -0.000000000000000000, -1.000000000000000000 ) ) ;
#9792=ORIENTED_EDGE ( 'NONE', *, *, #4801, .F. ) ;
#9807=AXIS2_PLACEMENT_3D ( 'NONE', #1522, #3258, #1568 ) ;
#9818=ORIENTED_EDGE ( 'NONE', *, *, #10466, .F. ) ;
#9822=DIRECTION ( 'NONE',  ( 0.000000000000000000, 1.000000000000000000, -0.000000000000000000 ) ) ;
#9833=UNCERTAINTY_MEASURE_WITH_UNIT (LENGTH_MEASURE( 1.000000000000000082E-05 ), #1764, 'distance_accuracy_value', 'NONE');
#9834=VERTEX_POINT ( 'NONE', #879 ) ;
#9873=VECTOR ( 'NONE', #1564, 1000.000000000000000 ) ;
#9890=EDGE_CURVE ( 'NONE', #7087, #2784, #6012, .T. ) ;
#9904=VECTOR ( 'NONE', #2467, 1000.000000000000000 ) ;
#9917=FACE_BOUND ( 'NONE', #1570, .T. ) ;
#9921=ADVANCED_FACE ( 'NONE', ( #6924 ), #10159, .F. ) ;
#9926=DIRECTION ( 'NONE',  ( -0.000000000000000000, -0.000000000000000000, 1.000000000000000000 ) ) ;
#9935=EDGE_CURVE ( 'NONE', #7686, #3419, #8335, .T. ) ;
#9943=MANIFOLD_SOLID_BREP ( 'Cut-Extrude9', #2494 ) ;
#9975=CIRCLE ( 'NONE', #325, 4.024999999999997691 ) ;
#9991=DIRECTION ( 'NONE',  ( 0.000000000000000000, 0.000000000000000000, -1.000000000000000000 ) ) ;
#9993=CARTESIAN_POINT ( 'NONE',  ( -11.29350689640809158, 105.5289575273812233, 7.749999999999999112 ) ) ;
#9996=CARTESIAN_POINT ( 'NONE',  ( -47.94539818030330025, 137.0132282531173473, 3.999999999999991562 ) ) ;
#10005=CARTESIAN_POINT ( 'NONE',  ( -56.34457570605425758, 137.0132282531173473, 0.000000000000000000 ) ) ;
#10007=DIRECTION ( 'NONE',  ( -0.000000000000000000, 0.000000000000000000, 1.000000000000000000 ) ) ;
#10010=FACE_OUTER_BOUND ( 'NONE', #9420, .T. ) ;
#10016=ADVANCED_FACE ( 'NONE', ( #445 ), #6285, .F. ) ;
#10018=CARTESIAN_POINT ( 'NONE',  ( -20.29350689640809691, 140.5696653505793563, 10.90000000000000036 ) ) ;
#10024=CARTESIAN_POINT ( 'NONE',  ( -3.173844575093148990, 150.5696653505793563, -10.90000000000000036 ) ) ;
#10040=EDGE_LOOP ( 'NONE', ( #8513, #6097, #3698, #2920, #1201 ) ) ;
#10043=ORIENTED_EDGE ( 'NONE', *, *, #3733, .T. ) ;
#10046=ORIENTED_EDGE ( 'NONE', *, *, #5206, .T. ) ;
#10051=CIRCLE ( 'NONE', #3274, 4.024999999999997691 ) ;
#10054=ORIENTED_EDGE ( 'NONE', *, *, #3911, .T. ) ;
#10058=CARTESIAN_POINT ( 'NONE',  ( -56.36957570605426326, 90.52895752738122326, 10.90000000000000036 ) ) ;
#10068=VECTOR ( 'NONE', #8926, 1000.000000000000000 ) ;
#10069=VERTEX_POINT ( 'NONE', #9397 ) ;
#10074=ADVANCED_FACE ( 'NONE', ( #6155, #6100, #9184 ), #5151, .F. ) ;
#10090=CARTESIAN_POINT ( 'NONE',  ( -55.94539818030328604, 145.0132282531173189, -3.999999999999992895 ) ) ;
#10118=CARTESIAN_POINT ( 'NONE',  ( 10.26554134690924691, 150.5696653505793563, 7.749999999999998224 ) ) ;
#10143=CARTESIAN_POINT ( 'NONE',  ( -47.94539818030330025, 90.52895752738122326, 3.999999999999993339 ) ) ;
#10149=EDGE_LOOP ( 'NONE', ( #7637, #8755, #5387, #6954 ) ) ;
#10155=EDGE_CURVE ( 'NONE', #7686, #382, #10158, .T. ) ;
#10158=( BOUNDED_CURVE ( )  B_SPLINE_CURVE ( 3, ( #6852, #10090, #6050, #11 ),
 .UNSPECIFIED., .F., .F. ) 
 B_SPLINE_CURVE_WITH_KNOTS ( ( 4, 4 ),
 ( 4.712388980384689674, 7.853981633974482790 ),
 .UNSPECIFIED. ) 
 CURVE ( )  GEOMETRIC_REPRESENTATION_ITEM ( )  RATIONAL_B_SPLINE_CURVE ( ( 1.000000000000000000, 0.3333333333333333703, 0.3333333333333333703, 1.000000000000000000 ) ) 
 REPRESENTATION_ITEM ( '' )  );
#10159=CYLINDRICAL_SURFACE ( 'NONE', #3932, 4.024999999999997691 ) ;
#10167=VERTEX_POINT ( 'NONE', #4038 ) ;
#10205=DIRECTION ( 'NONE',  ( 0.000000000000000000, 0.000000000000000000, 1.000000000000000000 ) ) ;
#10214=AXIS2_PLACEMENT_3D ( 'NONE', #435, #380, #6840 ) ;
#10229=CARTESIAN_POINT ( 'NONE',  ( -56.36957570605427037, 137.0132282531173473, -3.999999999999989786 ) ) ;
#10233=LINE ( 'NONE', #4452, #1466 ) ;
#10246=VERTEX_POINT ( 'NONE', #699 ) ;
#10249=AXIS2_PLACEMENT_3D ( 'NONE', #7678, #2794, #2903 ) ;
#10253=CARTESIAN_POINT ( 'NONE',  ( -27.85255513972543895, 64.37996872128307757, 7.750000000000002665 ) ) ;
#10256=VERTEX_POINT ( 'NONE', #4620 ) ;
#10259=LINE ( 'NONE', #2994, #6891 ) ;
#10267=ORIENTED_EDGE ( 'NONE', *, *, #1053, .T. ) ;
#10273=ORIENTED_EDGE ( 'NONE', *, *, #9501, .T. ) ;
#10277=VECTOR ( 'NONE', #6417, 1000.000000000000000 ) ;
#10283=EDGE_CURVE ( 'NONE', #6231, #3393, #10365, .T. ) ;
#10300=ORIENTED_EDGE ( 'NONE', *, *, #8186, .F. ) ;
#10325=CARTESIAN_POINT ( 'NONE',  ( -56.36957570605427748, 150.5696653505793563, 10.90000000000000036 ) ) ;
#10326=AXIS2_PLACEMENT_3D ( 'NONE', #2533, #6455, #3336 ) ;
#10330=DIRECTION ( 'NONE',  ( 0.000000000000000000, 0.000000000000000000, 1.000000000000000000 ) ) ;
#10363=FACE_BOUND ( 'NONE', #6887, .T. ) ;
#10365=CIRCLE ( 'NONE', #4928, 4.025000000000000355 ) ;
#10377=ORIENTED_EDGE ( 'NONE', *, *, #3719, .T. ) ;
#10393=DIRECTION ( 'NONE',  ( 1.000000000000000000, 0.000000000000000000, -2.154935995002246132E-16 ) ) ;
#10410=DIRECTION ( 'NONE',  ( 1.000000000000000000, 0.000000000000000000, 0.000000000000000000 ) ) ;
#10414=CARTESIAN_POINT ( 'NONE',  ( 10.26554134690924691, 64.37996872128307757, 7.749999999999998224 ) ) ;
#10419=VERTEX_POINT ( 'NONE', #3716 ) ;
#10427=EDGE_LOOP ( 'NONE', ( #7471, #10300 ) ) ;
#10457=CARTESIAN_POINT ( 'NONE',  ( -47.94539818030330025, 137.0132282531173473, 3.999999999999991562 ) ) ;
#10464=ADVANCED_FACE ( 'NONE', ( #4507 ), #3243, .F. ) ;
#10466=EDGE_CURVE ( 'NONE', #1746, #10256, #4095, .T. ) ;
#10474=AXIS2_PLACEMENT_3D ( 'NONE', #1685, #7305, #50 ) ;
#10526=COLOUR_RGB('Off White',0.89,0.88,0.83);
#10527=FILL_AREA_STYLE_COLOUR('',#10526);
#10528=FILL_AREA_STYLE('',(#10527));
#10529=SURFACE_STYLE_FILL_AREA(#10528);
#10530=SURFACE_SIDE_STYLE('',(#10529));
#10531=SURFACE_STYLE_USAGE(.BOTH.,#10530);
#10532=PRESENTATION_STYLE_ASSIGNMENT((#10531));
ENDSEC;
END-ISO-10303-21;
